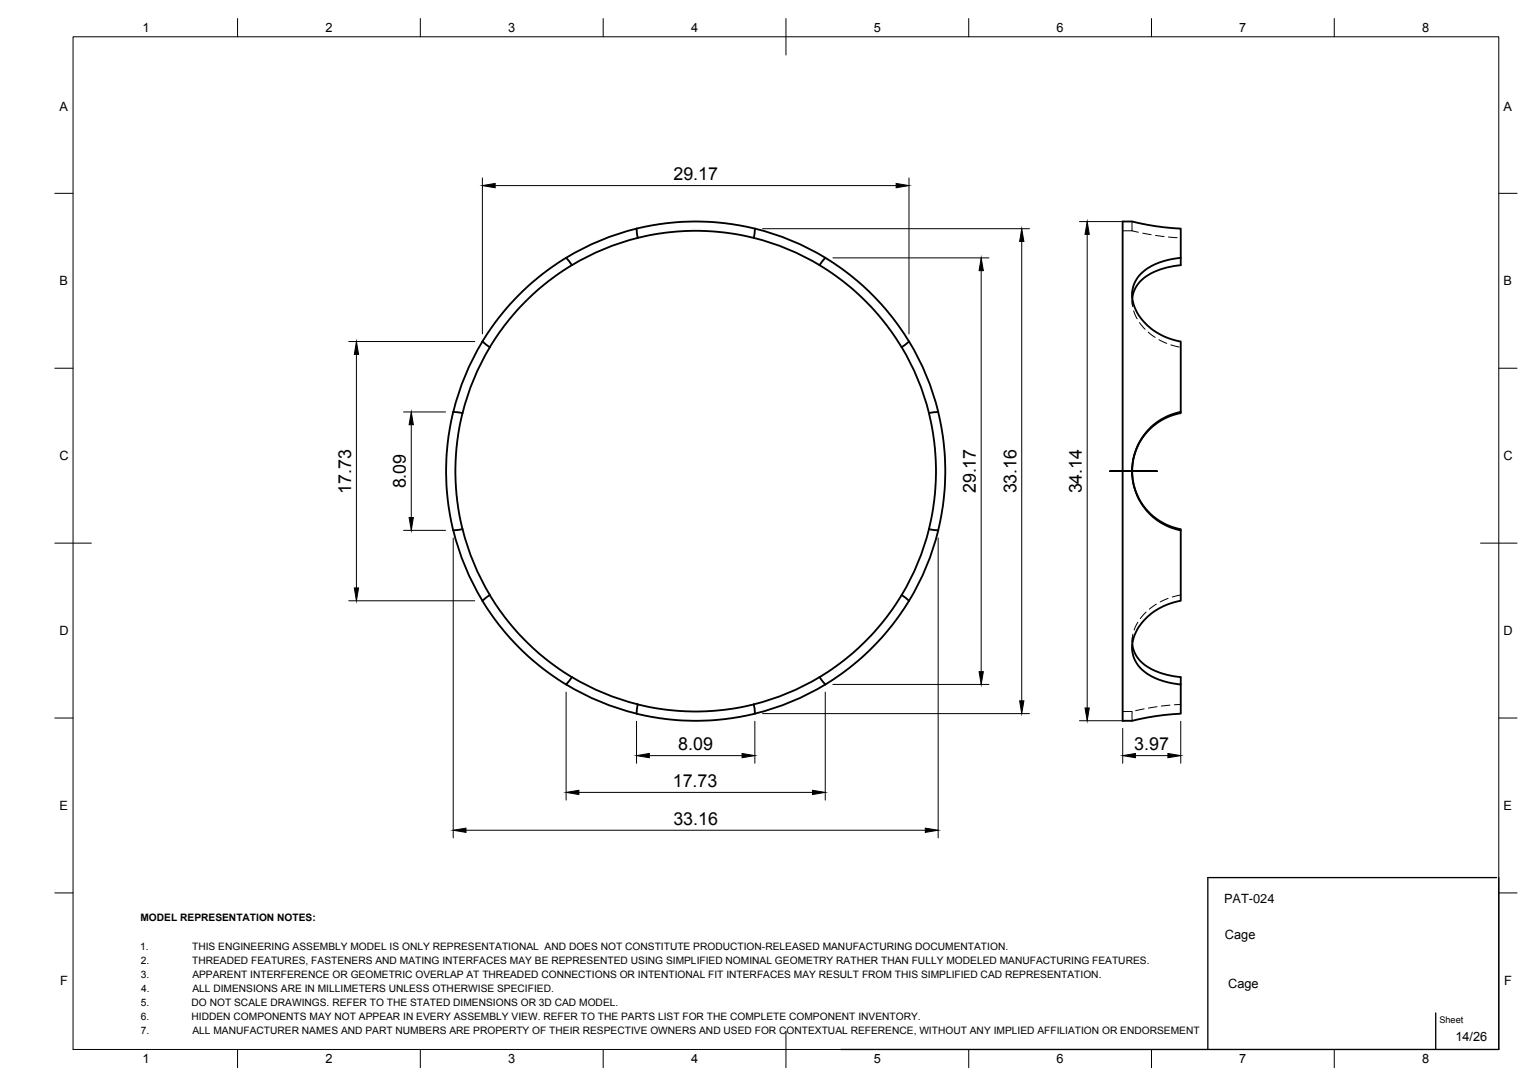
ISO-10303-21;
HEADER;
/* Generated by software containing ST-Developer
 * from STEP Tools, Inc. (www.steptools.com) 
 */

FILE_DESCRIPTION(
/* description */ ('Compact handwheel screw vise'),
/* implementation_level */ '2;1');

FILE_NAME(
/* name */ 'Cage.step',
/* time_stamp */ '2026-10-29T16:08:22-07:00',
/* author */ (''),
/* organization */ (''),
/* preprocessor_version */ 'ST-DEVELOPER v20.2',
/* originating_system */ 'Autodesk Translation Framework v15.17.0.0',
/* authorisation */ '');

FILE_SCHEMA (('AUTOMOTIVE_DESIGN { 1 0 10303 214 3 1 1 }'));
ENDSEC;

DATA;
#10=MECHANICAL_DESIGN_GEOMETRIC_PRESENTATION_REPRESENTATION('',(#661),#25074);
#211=B_SPLINE_CURVE_WITH_KNOTS('',3,(#11837,#11838,#11839,#11840,#11841,
#11842,#11843,#11844,#11845,#11846,#11847,#11848,#11849,#11850,#11851,#11852,
#11853,#11854,#11855,#11856,#11857,#11858),.UNSPECIFIED.,.F.,.F.,(4,2,2,
2,2,2,2,2,2,2,4),(0.0789094028588958,0.210573405340968,0.315860108011452,
0.421146810681936,0.522142632548711,0.623138454415485,0.72413427628226,
0.825130098149035,0.930416800819519,1.03570350349,1.16736750597208),
 .UNSPECIFIED.);
#212=B_SPLINE_CURVE_WITH_KNOTS('',3,(#11862,#11863,#11864,#11865,#11866,
#11867,#11868,#11869,#11870,#11871,#11872,#11873,#11874,#11875,#11876,#11877,
#11878,#11879,#11880,#11881,#11882,#11883),.UNSPECIFIED.,.F.,.F.,(4,2,2,
2,2,2,2,2,2,2,4),(0.0774793363974613,0.142088896491891,0.284177792983782,
0.411119756996526,0.514392970548519,0.617666184100513,0.720939397652506,
0.8242126112045,0.951154575217244,1.09324347170913,1.15785303180356),
 .UNSPECIFIED.);
#213=B_SPLINE_CURVE_WITH_KNOTS('',3,(#11889,#11890,#11891,#11892,#11893,
#11894,#11895,#11896,#11897,#11898,#11899,#11900,#11901,#11902,#11903,#11904,
#11905,#11906,#11907,#11908,#11909,#11910),.UNSPECIFIED.,.F.,.F.,(4,2,2,
2,2,2,2,2,2,2,4),(0.0774793363974613,0.142088896491891,0.284177792983782,
0.411119756996525,0.514392970548519,0.617666184100513,0.720939397652506,
0.8242126112045,0.951154575217243,1.09324347170913,1.15785303180356),
 .UNSPECIFIED.);
#214=B_SPLINE_CURVE_WITH_KNOTS('',3,(#11914,#11915,#11916,#11917,#11918,
#11919,#11920,#11921,#11922,#11923,#11924,#11925,#11926,#11927,#11928,#11929,
#11930,#11931,#11932,#11933,#11934,#11935),.UNSPECIFIED.,.F.,.F.,(4,2,2,
2,2,2,2,2,2,2,4),(0.0774793363974614,0.142088896491891,0.284177792983781,
0.411119756996525,0.514392970548519,0.617666184100512,0.720939397652506,
0.824212611204499,0.951154575217243,1.09324347170913,1.15785303180356),
 .UNSPECIFIED.);
#215=B_SPLINE_CURVE_WITH_KNOTS('',3,(#11939,#11940,#11941,#11942,#11943,
#11944,#11945,#11946,#11947,#11948,#11949,#11950),.UNSPECIFIED.,.F.,.F.,
(4,2,2,2,2,4),(0.0774793363974613,0.142088896491891,0.284177792983781,0.411119756996525,
0.514392970548519,0.617666184100512),.UNSPECIFIED.);
#216=B_SPLINE_CURVE_WITH_KNOTS('',3,(#11955,#11956,#11957,#11958,#11959,
#11960,#11961,#11962,#11963,#11964,#11965,#11966),.UNSPECIFIED.,.F.,.F.,
(4,2,2,2,2,4),(0.617666184100512,0.720939397652506,0.824212611204499,0.951154575217243,
1.09324347170913,1.15785303180356),.UNSPECIFIED.);
#217=B_SPLINE_CURVE_WITH_KNOTS('',3,(#11970,#11971,#11972,#11973,#11974,
#11975,#11976,#11977,#11978,#11979,#11980,#11981,#11982,#11983,#11984,#11985,
#11986,#11987,#11988,#11989,#11990,#11991),.UNSPECIFIED.,.F.,.F.,(4,2,2,
2,2,2,2,2,2,2,4),(0.0774793363974613,0.142088896491891,0.284177792983782,
0.411119756996526,0.514392970548519,0.617666184100513,0.720939397652507,
0.8242126112045,0.951154575217245,1.09324347170914,1.15785303180356),
 .UNSPECIFIED.);
#218=B_SPLINE_CURVE_WITH_KNOTS('',3,(#11995,#11996,#11997,#11998,#11999,
#12000,#12001,#12002,#12003,#12004,#12005,#12006,#12007,#12008,#12009,#12010,
#12011,#12012,#12013,#12014,#12015,#12016),.UNSPECIFIED.,.F.,.F.,(4,2,2,
2,2,2,2,2,2,2,4),(0.0774793363974613,0.142088896491891,0.284177792983782,
0.411119756996526,0.514392970548519,0.617666184100513,0.720939397652506,
0.824212611204499,0.951154575217243,1.09324347170913,1.15785303180356),
 .UNSPECIFIED.);
#219=B_SPLINE_CURVE_WITH_KNOTS('',3,(#12020,#12021,#12022,#12023,#12024,
#12025,#12026,#12027,#12028,#12029,#12030,#12031,#12032,#12033,#12034,#12035,
#12036,#12037,#12038,#12039,#12040,#12041),.UNSPECIFIED.,.F.,.F.,(4,2,2,
2,2,2,2,2,2,2,4),(0.0774793363974613,0.142088896491891,0.284177792983782,
0.411119756996526,0.514392970548519,0.617666184100513,0.720939397652506,
0.8242126112045,0.951154575217244,1.09324347170913,1.15785303180356),
 .UNSPECIFIED.);
#220=B_SPLINE_CURVE_WITH_KNOTS('',3,(#12045,#12046,#12047,#12048,#12049,
#12050,#12051,#12052,#12053,#12054,#12055,#12056,#12057,#12058,#12059,#12060,
#12061,#12062,#12063,#12064,#12065,#12066),.UNSPECIFIED.,.F.,.F.,(4,2,2,
2,2,2,2,2,2,2,4),(0.0774793363974613,0.142088896491891,0.284177792983782,
0.411119756996526,0.514392970548519,0.617666184100513,0.720939397652506,
0.8242126112045,0.951154575217243,1.09324347170913,1.15785303180356),
 .UNSPECIFIED.);
#221=B_SPLINE_CURVE_WITH_KNOTS('',3,(#12074,#12075,#12076,#12077,#12078,
#12079,#12080,#12081,#12082,#12083,#12084,#12085,#12086,#12087,#12088,#12089,
#12090,#12091,#12092,#12093,#12094,#12095),.UNSPECIFIED.,.F.,.F.,(4,2,2,
2,2,2,2,2,2,2,4),(0.0789094028588958,0.210573405340968,0.315860108011452,
0.421146810681936,0.522142632548711,0.623138454415485,0.72413427628226,
0.825130098149035,0.930416800819519,1.03570350349,1.16736750597208),
 .UNSPECIFIED.);
#222=B_SPLINE_CURVE_WITH_KNOTS('',3,(#12103,#12104,#12105,#12106,#12107,
#12108,#12109,#12110,#12111,#12112,#12113,#12114,#12115,#12116,#12117,#12118,
#12119,#12120,#12121,#12122,#12123,#12124),.UNSPECIFIED.,.F.,.F.,(4,2,2,
2,2,2,2,2,2,2,4),(0.0789094028588958,0.210573405340969,0.315860108011453,
0.421146810681937,0.522142632548712,0.623138454415486,0.724134276282261,
0.825130098149035,0.930416800819519,1.03570350349,1.16736750597208),
 .UNSPECIFIED.);
#223=B_SPLINE_CURVE_WITH_KNOTS('',3,(#12133,#12134,#12135,#12136,#12137,
#12138,#12139,#12140,#12141,#12142,#12143,#12144),.UNSPECIFIED.,.F.,.F.,
(4,2,2,2,2,4),(0.0789094028588958,0.210573405340968,0.315860108011452,0.421146810681937,
0.522142632548711,0.623138454415486),.UNSPECIFIED.);
#224=B_SPLINE_CURVE_WITH_KNOTS('',3,(#12146,#12147,#12148,#12149,#12150,
#12151,#12152,#12153,#12154,#12155,#12156,#12157),.UNSPECIFIED.,.F.,.F.,
(4,2,2,2,2,4),(0.623138454415486,0.72413427628226,0.825130098149035,0.930416800819519,
1.03570350349,1.16736750597208),.UNSPECIFIED.);
#225=B_SPLINE_CURVE_WITH_KNOTS('',3,(#12164,#12165,#12166,#12167,#12168,
#12169,#12170,#12171,#12172,#12173,#12174,#12175,#12176,#12177,#12178,#12179,
#12180,#12181,#12182,#12183,#12184,#12185),.UNSPECIFIED.,.F.,.F.,(4,2,2,
2,2,2,2,2,2,2,4),(0.0789094028588958,0.210573405340968,0.315860108011452,
0.421146810681936,0.522142632548711,0.623138454415486,0.72413427628226,
0.825130098149035,0.930416800819519,1.03570350349,1.16736750597208),
 .UNSPECIFIED.);
#226=B_SPLINE_CURVE_WITH_KNOTS('',3,(#12193,#12194,#12195,#12196,#12197,
#12198,#12199,#12200,#12201,#12202,#12203,#12204,#12205,#12206,#12207,#12208,
#12209,#12210,#12211,#12212,#12213,#12214),.UNSPECIFIED.,.F.,.F.,(4,2,2,
2,2,2,2,2,2,2,4),(0.0789094028588957,0.210573405340968,0.315860108011452,
0.421146810681936,0.522142632548711,0.623138454415485,0.72413427628226,
0.825130098149035,0.930416800819519,1.03570350349,1.16736750597207),
 .UNSPECIFIED.);
#227=B_SPLINE_CURVE_WITH_KNOTS('',3,(#12222,#12223,#12224,#12225,#12226,
#12227,#12228,#12229,#12230,#12231,#12232,#12233,#12234,#12235,#12236,#12237,
#12238,#12239,#12240,#12241,#12242,#12243),.UNSPECIFIED.,.F.,.F.,(4,2,2,
2,2,2,2,2,2,2,4),(0.0789094028588958,0.210573405340968,0.315860108011452,
0.421146810681936,0.522142632548711,0.623138454415486,0.72413427628226,
0.825130098149035,0.930416800819519,1.03570350349,1.16736750597208),
 .UNSPECIFIED.);
#228=B_SPLINE_CURVE_WITH_KNOTS('',3,(#12252,#12253,#12254,#12255,#12256,
#12257,#12258,#12259,#12260,#12261,#12262,#12263,#12264,#12265,#12266,#12267,
#12268,#12269,#12270,#12271,#12272,#12273),.UNSPECIFIED.,.F.,.F.,(4,2,2,
2,2,2,2,2,2,2,4),(0.0789094028588958,0.210573405340968,0.315860108011452,
0.421146810681936,0.522142632548711,0.623138454415485,0.72413427628226,
0.825130098149035,0.930416800819519,1.03570350349,1.16736750597208),
 .UNSPECIFIED.);
#549=SPHERICAL_SURFACE('',#8631,0.412776);
#550=SPHERICAL_SURFACE('',#8647,0.412776);
#551=SPHERICAL_SURFACE('',#8652,0.412776);
#552=SPHERICAL_SURFACE('',#8657,0.412776);
#553=SPHERICAL_SURFACE('',#8662,0.412776);
#554=SPHERICAL_SURFACE('',#8667,0.412776);
#555=SPHERICAL_SURFACE('',#8672,0.412776);
#556=SPHERICAL_SURFACE('',#8680,0.412776);
#598=SHAPE_REPRESENTATION_RELATIONSHIP('SRR','None',#25207,#626);
#626=ADVANCED_BREP_SHAPE_REPRESENTATION('',(#696),#25054);
#661=STYLED_ITEM('',(#25439),#696);
#696=MANIFOLD_SOLID_BREP('Continuous crown cage',#8070);
#764=FACE_BOUND('',#1669,.T.);
#883=PLANE('',#8644);
#884=PLANE('',#8649);
#885=PLANE('',#8654);
#886=PLANE('',#8659);
#887=PLANE('',#8664);
#888=PLANE('',#8669);
#889=PLANE('',#8678);
#890=PLANE('',#8682);
#891=PLANE('',#8683);
#1129=FACE_OUTER_BOUND('',#1651,.T.);
#1130=FACE_OUTER_BOUND('',#1652,.T.);
#1131=FACE_OUTER_BOUND('',#1653,.T.);
#1132=FACE_OUTER_BOUND('',#1654,.T.);
#1133=FACE_OUTER_BOUND('',#1655,.T.);
#1134=FACE_OUTER_BOUND('',#1656,.T.);
#1135=FACE_OUTER_BOUND('',#1657,.T.);
#1136=FACE_OUTER_BOUND('',#1658,.T.);
#1137=FACE_OUTER_BOUND('',#1659,.T.);
#1138=FACE_OUTER_BOUND('',#1660,.T.);
#1139=FACE_OUTER_BOUND('',#1661,.T.);
#1140=FACE_OUTER_BOUND('',#1662,.T.);
#1141=FACE_OUTER_BOUND('',#1663,.T.);
#1142=FACE_OUTER_BOUND('',#1664,.T.);
#1143=FACE_OUTER_BOUND('',#1665,.T.);
#1144=FACE_OUTER_BOUND('',#1666,.T.);
#1145=FACE_OUTER_BOUND('',#1667,.T.);
#1146=FACE_OUTER_BOUND('',#1668,.T.);
#1147=FACE_OUTER_BOUND('',#1670,.T.);
#1651=EDGE_LOOP('',(#5611,#5612,#5613,#5614));
#1652=EDGE_LOOP('',(#5615,#5616,#5617,#5618,#5619,#5620,#5621,#5622,#5623,
#5624,#5625,#5626,#5627,#5628,#5629,#5630,#5631,#5632,#5633,#5634));
#1653=EDGE_LOOP('',(#5635,#5636,#5637,#5638));
#1654=EDGE_LOOP('',(#5639,#5640,#5641,#5642));
#1655=EDGE_LOOP('',(#5643,#5644,#5645,#5646));
#1656=EDGE_LOOP('',(#5647,#5648,#5649,#5650));
#1657=EDGE_LOOP('',(#5651,#5652,#5653,#5654));
#1658=EDGE_LOOP('',(#5655,#5656,#5657,#5658,#5659,#5660));
#1659=EDGE_LOOP('',(#5661,#5662,#5663,#5664));
#1660=EDGE_LOOP('',(#5665,#5666,#5667,#5668));
#1661=EDGE_LOOP('',(#5669,#5670,#5671,#5672));
#1662=EDGE_LOOP('',(#5673,#5674,#5675,#5676));
#1663=EDGE_LOOP('',(#5677,#5678,#5679,#5680));
#1664=EDGE_LOOP('',(#5681,#5682,#5683,#5684));
#1665=EDGE_LOOP('',(#5685,#5686,#5687,#5688,#5689,#5690,#5691,#5692,#5693,
#5694,#5695,#5696,#5697,#5698,#5699,#5700,#5701,#5702,#5703,#5704));
#1666=EDGE_LOOP('',(#5705,#5706,#5707,#5708));
#1667=EDGE_LOOP('',(#5709,#5710,#5711,#5712));
#1668=EDGE_LOOP('',(#5713));
#1669=EDGE_LOOP('',(#5714));
#1670=EDGE_LOOP('',(#5715,#5716,#5717,#5718));
#2189=LINE('',#11952,#2697);
#2190=LINE('',#12248,#2698);
#2697=VECTOR('',#9805,1.706752);
#2698=VECTOR('',#9882,1.643248);
#3177=CIRCLE('',#8632,0.405071403305639);
#3178=CIRCLE('',#8633,0.405071403305639);
#3179=CIRCLE('',#8635,1.706752);
#3180=CIRCLE('',#8636,1.706752);
#3181=CIRCLE('',#8637,1.706752);
#3182=CIRCLE('',#8638,1.706752);
#3183=CIRCLE('',#8639,1.706752);
#3184=CIRCLE('',#8640,1.706752);
#3185=CIRCLE('',#8641,1.706752);
#3186=CIRCLE('',#8642,1.706752);
#3187=CIRCLE('',#8643,1.706752);
#3188=CIRCLE('',#8645,1.643248);
#3189=CIRCLE('',#8646,0.405071403305639);
#3190=CIRCLE('',#8648,0.405071403305639);
#3191=CIRCLE('',#8650,1.643248);
#3192=CIRCLE('',#8651,0.405071403305639);
#3193=CIRCLE('',#8653,0.405071403305639);
#3194=CIRCLE('',#8655,1.643248);
#3195=CIRCLE('',#8656,0.405071403305639);
#3196=CIRCLE('',#8658,0.405071403305639);
#3197=CIRCLE('',#8660,1.643248);
#3198=CIRCLE('',#8661,0.405071403305639);
#3199=CIRCLE('',#8663,0.405071403305639);
#3200=CIRCLE('',#8665,1.643248);
#3201=CIRCLE('',#8666,0.405071403305639);
#3202=CIRCLE('',#8668,0.405071403305639);
#3203=CIRCLE('',#8670,1.643248);
#3204=CIRCLE('',#8671,0.405071403305639);
#3205=CIRCLE('',#8673,0.405071403305639);
#3206=CIRCLE('',#8675,1.643248);
#3207=CIRCLE('',#8676,1.643248);
#3208=CIRCLE('',#8677,1.643248);
#3209=CIRCLE('',#8679,0.405071403305639);
#3210=CIRCLE('',#8681,0.405071403305639);
#3492=VERTEX_POINT('',#11835);
#3493=VERTEX_POINT('',#11836);
#3494=VERTEX_POINT('',#11859);
#3495=VERTEX_POINT('',#11861);
#3496=VERTEX_POINT('',#11886);
#3497=VERTEX_POINT('',#11888);
#3498=VERTEX_POINT('',#11911);
#3499=VERTEX_POINT('',#11913);
#3500=VERTEX_POINT('',#11936);
#3501=VERTEX_POINT('',#11938);
#3502=VERTEX_POINT('',#11951);
#3503=VERTEX_POINT('',#11954);
#3504=VERTEX_POINT('',#11967);
#3505=VERTEX_POINT('',#11969);
#3506=VERTEX_POINT('',#11992);
#3507=VERTEX_POINT('',#11994);
#3508=VERTEX_POINT('',#12017);
#3509=VERTEX_POINT('',#12019);
#3510=VERTEX_POINT('',#12042);
#3511=VERTEX_POINT('',#12044);
#3512=VERTEX_POINT('',#12069);
#3513=VERTEX_POINT('',#12073);
#3514=VERTEX_POINT('',#12098);
#3515=VERTEX_POINT('',#12102);
#3516=VERTEX_POINT('',#12127);
#3517=VERTEX_POINT('',#12131);
#3518=VERTEX_POINT('',#12132);
#3519=VERTEX_POINT('',#12159);
#3520=VERTEX_POINT('',#12163);
#3521=VERTEX_POINT('',#12188);
#3522=VERTEX_POINT('',#12192);
#3523=VERTEX_POINT('',#12217);
#3524=VERTEX_POINT('',#12221);
#3525=VERTEX_POINT('',#12246);
#3526=VERTEX_POINT('',#12249);
#3527=VERTEX_POINT('',#12251);
#4292=EDGE_CURVE('',#3492,#3493,#211,.T.);
#4293=EDGE_CURVE('',#3494,#3492,#3177,.T.);
#4294=EDGE_CURVE('',#3495,#3494,#212,.T.);
#4295=EDGE_CURVE('',#3493,#3495,#3178,.T.);
#4296=EDGE_CURVE('',#3496,#3494,#3179,.T.);
#4297=EDGE_CURVE('',#3496,#3497,#213,.T.);
#4298=EDGE_CURVE('',#3498,#3497,#3180,.T.);
#4299=EDGE_CURVE('',#3498,#3499,#214,.T.);
#4300=EDGE_CURVE('',#3500,#3499,#3181,.T.);
#4301=EDGE_CURVE('',#3500,#3501,#215,.T.);
#4302=EDGE_CURVE('',#3501,#3502,#2189,.T.);
#4303=EDGE_CURVE('',#3502,#3502,#3182,.T.);
#4304=EDGE_CURVE('',#3501,#3503,#216,.T.);
#4305=EDGE_CURVE('',#3504,#3503,#3183,.T.);
#4306=EDGE_CURVE('',#3504,#3505,#217,.T.);
#4307=EDGE_CURVE('',#3506,#3505,#3184,.T.);
#4308=EDGE_CURVE('',#3506,#3507,#218,.T.);
#4309=EDGE_CURVE('',#3508,#3507,#3185,.T.);
#4310=EDGE_CURVE('',#3508,#3509,#219,.T.);
#4311=EDGE_CURVE('',#3510,#3509,#3186,.T.);
#4312=EDGE_CURVE('',#3510,#3511,#220,.T.);
#4313=EDGE_CURVE('',#3495,#3511,#3187,.T.);
#4314=EDGE_CURVE('',#3492,#3512,#3188,.T.);
#4315=EDGE_CURVE('',#3512,#3496,#3189,.T.);
#4316=EDGE_CURVE('',#3513,#3512,#221,.T.);
#4317=EDGE_CURVE('',#3497,#3513,#3190,.T.);
#4318=EDGE_CURVE('',#3513,#3514,#3191,.T.);
#4319=EDGE_CURVE('',#3514,#3498,#3192,.T.);
#4320=EDGE_CURVE('',#3515,#3514,#222,.T.);
#4321=EDGE_CURVE('',#3499,#3515,#3193,.T.);
#4322=EDGE_CURVE('',#3515,#3516,#3194,.T.);
#4323=EDGE_CURVE('',#3516,#3500,#3195,.T.);
#4324=EDGE_CURVE('',#3517,#3518,#223,.T.);
#4325=EDGE_CURVE('',#3503,#3517,#3196,.T.);
#4326=EDGE_CURVE('',#3518,#3516,#224,.T.);
#4327=EDGE_CURVE('',#3517,#3519,#3197,.T.);
#4328=EDGE_CURVE('',#3519,#3504,#3198,.T.);
#4329=EDGE_CURVE('',#3520,#3519,#225,.T.);
#4330=EDGE_CURVE('',#3505,#3520,#3199,.T.);
#4331=EDGE_CURVE('',#3520,#3521,#3200,.T.);
#4332=EDGE_CURVE('',#3521,#3506,#3201,.T.);
#4333=EDGE_CURVE('',#3522,#3521,#226,.T.);
#4334=EDGE_CURVE('',#3507,#3522,#3202,.T.);
#4335=EDGE_CURVE('',#3522,#3523,#3203,.T.);
#4336=EDGE_CURVE('',#3523,#3508,#3204,.T.);
#4337=EDGE_CURVE('',#3524,#3523,#227,.T.);
#4338=EDGE_CURVE('',#3509,#3524,#3205,.T.);
#4339=EDGE_CURVE('',#3525,#3525,#3206,.T.);
#4340=EDGE_CURVE('',#3525,#3518,#2190,.T.);
#4341=EDGE_CURVE('',#3526,#3493,#3207,.T.);
#4342=EDGE_CURVE('',#3526,#3527,#228,.T.);
#4343=EDGE_CURVE('',#3524,#3527,#3208,.T.);
#4344=EDGE_CURVE('',#3511,#3526,#3209,.T.);
#4345=EDGE_CURVE('',#3527,#3510,#3210,.T.);
#5611=ORIENTED_EDGE('',*,*,#4292,.F.);
#5612=ORIENTED_EDGE('',*,*,#4293,.F.);
#5613=ORIENTED_EDGE('',*,*,#4294,.F.);
#5614=ORIENTED_EDGE('',*,*,#4295,.F.);
#5615=ORIENTED_EDGE('',*,*,#4294,.T.);
#5616=ORIENTED_EDGE('',*,*,#4296,.F.);
#5617=ORIENTED_EDGE('',*,*,#4297,.T.);
#5618=ORIENTED_EDGE('',*,*,#4298,.F.);
#5619=ORIENTED_EDGE('',*,*,#4299,.T.);
#5620=ORIENTED_EDGE('',*,*,#4300,.F.);
#5621=ORIENTED_EDGE('',*,*,#4301,.T.);
#5622=ORIENTED_EDGE('',*,*,#4302,.T.);
#5623=ORIENTED_EDGE('',*,*,#4303,.F.);
#5624=ORIENTED_EDGE('',*,*,#4302,.F.);
#5625=ORIENTED_EDGE('',*,*,#4304,.T.);
#5626=ORIENTED_EDGE('',*,*,#4305,.F.);
#5627=ORIENTED_EDGE('',*,*,#4306,.T.);
#5628=ORIENTED_EDGE('',*,*,#4307,.F.);
#5629=ORIENTED_EDGE('',*,*,#4308,.T.);
#5630=ORIENTED_EDGE('',*,*,#4309,.F.);
#5631=ORIENTED_EDGE('',*,*,#4310,.T.);
#5632=ORIENTED_EDGE('',*,*,#4311,.F.);
#5633=ORIENTED_EDGE('',*,*,#4312,.T.);
#5634=ORIENTED_EDGE('',*,*,#4313,.F.);
#5635=ORIENTED_EDGE('',*,*,#4293,.T.);
#5636=ORIENTED_EDGE('',*,*,#4314,.T.);
#5637=ORIENTED_EDGE('',*,*,#4315,.T.);
#5638=ORIENTED_EDGE('',*,*,#4296,.T.);
#5639=ORIENTED_EDGE('',*,*,#4316,.F.);
#5640=ORIENTED_EDGE('',*,*,#4317,.F.);
#5641=ORIENTED_EDGE('',*,*,#4297,.F.);
#5642=ORIENTED_EDGE('',*,*,#4315,.F.);
#5643=ORIENTED_EDGE('',*,*,#4317,.T.);
#5644=ORIENTED_EDGE('',*,*,#4318,.T.);
#5645=ORIENTED_EDGE('',*,*,#4319,.T.);
#5646=ORIENTED_EDGE('',*,*,#4298,.T.);
#5647=ORIENTED_EDGE('',*,*,#4320,.F.);
#5648=ORIENTED_EDGE('',*,*,#4321,.F.);
#5649=ORIENTED_EDGE('',*,*,#4299,.F.);
#5650=ORIENTED_EDGE('',*,*,#4319,.F.);
#5651=ORIENTED_EDGE('',*,*,#4321,.T.);
#5652=ORIENTED_EDGE('',*,*,#4322,.T.);
#5653=ORIENTED_EDGE('',*,*,#4323,.T.);
#5654=ORIENTED_EDGE('',*,*,#4300,.T.);
#5655=ORIENTED_EDGE('',*,*,#4324,.F.);
#5656=ORIENTED_EDGE('',*,*,#4325,.F.);
#5657=ORIENTED_EDGE('',*,*,#4304,.F.);
#5658=ORIENTED_EDGE('',*,*,#4301,.F.);
#5659=ORIENTED_EDGE('',*,*,#4323,.F.);
#5660=ORIENTED_EDGE('',*,*,#4326,.F.);
#5661=ORIENTED_EDGE('',*,*,#4325,.T.);
#5662=ORIENTED_EDGE('',*,*,#4327,.T.);
#5663=ORIENTED_EDGE('',*,*,#4328,.T.);
#5664=ORIENTED_EDGE('',*,*,#4305,.T.);
#5665=ORIENTED_EDGE('',*,*,#4329,.F.);
#5666=ORIENTED_EDGE('',*,*,#4330,.F.);
#5667=ORIENTED_EDGE('',*,*,#4306,.F.);
#5668=ORIENTED_EDGE('',*,*,#4328,.F.);
#5669=ORIENTED_EDGE('',*,*,#4330,.T.);
#5670=ORIENTED_EDGE('',*,*,#4331,.T.);
#5671=ORIENTED_EDGE('',*,*,#4332,.T.);
#5672=ORIENTED_EDGE('',*,*,#4307,.T.);
#5673=ORIENTED_EDGE('',*,*,#4333,.F.);
#5674=ORIENTED_EDGE('',*,*,#4334,.F.);
#5675=ORIENTED_EDGE('',*,*,#4308,.F.);
#5676=ORIENTED_EDGE('',*,*,#4332,.F.);
#5677=ORIENTED_EDGE('',*,*,#4334,.T.);
#5678=ORIENTED_EDGE('',*,*,#4335,.T.);
#5679=ORIENTED_EDGE('',*,*,#4336,.T.);
#5680=ORIENTED_EDGE('',*,*,#4309,.T.);
#5681=ORIENTED_EDGE('',*,*,#4310,.F.);
#5682=ORIENTED_EDGE('',*,*,#4336,.F.);
#5683=ORIENTED_EDGE('',*,*,#4337,.F.);
#5684=ORIENTED_EDGE('',*,*,#4338,.F.);
#5685=ORIENTED_EDGE('',*,*,#4339,.F.);
#5686=ORIENTED_EDGE('',*,*,#4340,.T.);
#5687=ORIENTED_EDGE('',*,*,#4326,.T.);
#5688=ORIENTED_EDGE('',*,*,#4322,.F.);
#5689=ORIENTED_EDGE('',*,*,#4320,.T.);
#5690=ORIENTED_EDGE('',*,*,#4318,.F.);
#5691=ORIENTED_EDGE('',*,*,#4316,.T.);
#5692=ORIENTED_EDGE('',*,*,#4314,.F.);
#5693=ORIENTED_EDGE('',*,*,#4292,.T.);
#5694=ORIENTED_EDGE('',*,*,#4341,.F.);
#5695=ORIENTED_EDGE('',*,*,#4342,.T.);
#5696=ORIENTED_EDGE('',*,*,#4343,.F.);
#5697=ORIENTED_EDGE('',*,*,#4337,.T.);
#5698=ORIENTED_EDGE('',*,*,#4335,.F.);
#5699=ORIENTED_EDGE('',*,*,#4333,.T.);
#5700=ORIENTED_EDGE('',*,*,#4331,.F.);
#5701=ORIENTED_EDGE('',*,*,#4329,.T.);
#5702=ORIENTED_EDGE('',*,*,#4327,.F.);
#5703=ORIENTED_EDGE('',*,*,#4324,.T.);
#5704=ORIENTED_EDGE('',*,*,#4340,.F.);
#5705=ORIENTED_EDGE('',*,*,#4295,.T.);
#5706=ORIENTED_EDGE('',*,*,#4313,.T.);
#5707=ORIENTED_EDGE('',*,*,#4344,.T.);
#5708=ORIENTED_EDGE('',*,*,#4341,.T.);
#5709=ORIENTED_EDGE('',*,*,#4312,.F.);
#5710=ORIENTED_EDGE('',*,*,#4345,.F.);
#5711=ORIENTED_EDGE('',*,*,#4342,.F.);
#5712=ORIENTED_EDGE('',*,*,#4344,.F.);
#5713=ORIENTED_EDGE('',*,*,#4303,.T.);
#5714=ORIENTED_EDGE('',*,*,#4339,.T.);
#5715=ORIENTED_EDGE('',*,*,#4338,.T.);
#5716=ORIENTED_EDGE('',*,*,#4343,.T.);
#5717=ORIENTED_EDGE('',*,*,#4345,.T.);
#5718=ORIENTED_EDGE('',*,*,#4311,.T.);
#7384=CYLINDRICAL_SURFACE('',#8634,1.706752);
#7385=CYLINDRICAL_SURFACE('',#8674,1.643248);
#7699=ADVANCED_FACE('',(#1129),#549,.F.);
#7700=ADVANCED_FACE('',(#1130),#7384,.T.);
#7701=ADVANCED_FACE('',(#1131),#883,.T.);
#7702=ADVANCED_FACE('',(#1132),#550,.F.);
#7703=ADVANCED_FACE('',(#1133),#884,.T.);
#7704=ADVANCED_FACE('',(#1134),#551,.F.);
#7705=ADVANCED_FACE('',(#1135),#885,.T.);
#7706=ADVANCED_FACE('',(#1136),#552,.F.);
#7707=ADVANCED_FACE('',(#1137),#886,.T.);
#7708=ADVANCED_FACE('',(#1138),#553,.F.);
#7709=ADVANCED_FACE('',(#1139),#887,.T.);
#7710=ADVANCED_FACE('',(#1140),#554,.F.);
#7711=ADVANCED_FACE('',(#1141),#888,.T.);
#7712=ADVANCED_FACE('',(#1142),#555,.F.);
#7713=ADVANCED_FACE('',(#1143),#7385,.F.);
#7714=ADVANCED_FACE('',(#1144),#889,.T.);
#7715=ADVANCED_FACE('',(#1145),#556,.F.);
#7716=ADVANCED_FACE('',(#1146,#764),#890,.T.);
#7717=ADVANCED_FACE('',(#1147),#891,.T.);
#8070=CLOSED_SHELL('',(#7699,#7700,#7701,#7702,#7703,#7704,#7705,#7706,
#7707,#7708,#7709,#7710,#7711,#7712,#7713,#7714,#7715,#7716,#7717));
#8630=AXIS2_PLACEMENT_3D('',#11833,#9789,#9790);
#8631=AXIS2_PLACEMENT_3D('',#11834,#9791,#9792);
#8632=AXIS2_PLACEMENT_3D('',#11860,#9793,#9794);
#8633=AXIS2_PLACEMENT_3D('',#11884,#9795,#9796);
#8634=AXIS2_PLACEMENT_3D('',#11885,#9797,#9798);
#8635=AXIS2_PLACEMENT_3D('',#11887,#9799,#9800);
#8636=AXIS2_PLACEMENT_3D('',#11912,#9801,#9802);
#8637=AXIS2_PLACEMENT_3D('',#11937,#9803,#9804);
#8638=AXIS2_PLACEMENT_3D('',#11953,#9806,#9807);
#8639=AXIS2_PLACEMENT_3D('',#11968,#9808,#9809);
#8640=AXIS2_PLACEMENT_3D('',#11993,#9810,#9811);
#8641=AXIS2_PLACEMENT_3D('',#12018,#9812,#9813);
#8642=AXIS2_PLACEMENT_3D('',#12043,#9814,#9815);
#8643=AXIS2_PLACEMENT_3D('',#12067,#9816,#9817);
#8644=AXIS2_PLACEMENT_3D('',#12068,#9818,#9819);
#8645=AXIS2_PLACEMENT_3D('',#12070,#9820,#9821);
#8646=AXIS2_PLACEMENT_3D('',#12071,#9822,#9823);
#8647=AXIS2_PLACEMENT_3D('',#12072,#9824,#9825);
#8648=AXIS2_PLACEMENT_3D('',#12096,#9826,#9827);
#8649=AXIS2_PLACEMENT_3D('',#12097,#9828,#9829);
#8650=AXIS2_PLACEMENT_3D('',#12099,#9830,#9831);
#8651=AXIS2_PLACEMENT_3D('',#12100,#9832,#9833);
#8652=AXIS2_PLACEMENT_3D('',#12101,#9834,#9835);
#8653=AXIS2_PLACEMENT_3D('',#12125,#9836,#9837);
#8654=AXIS2_PLACEMENT_3D('',#12126,#9838,#9839);
#8655=AXIS2_PLACEMENT_3D('',#12128,#9840,#9841);
#8656=AXIS2_PLACEMENT_3D('',#12129,#9842,#9843);
#8657=AXIS2_PLACEMENT_3D('',#12130,#9844,#9845);
#8658=AXIS2_PLACEMENT_3D('',#12145,#9846,#9847);
#8659=AXIS2_PLACEMENT_3D('',#12158,#9848,#9849);
#8660=AXIS2_PLACEMENT_3D('',#12160,#9850,#9851);
#8661=AXIS2_PLACEMENT_3D('',#12161,#9852,#9853);
#8662=AXIS2_PLACEMENT_3D('',#12162,#9854,#9855);
#8663=AXIS2_PLACEMENT_3D('',#12186,#9856,#9857);
#8664=AXIS2_PLACEMENT_3D('',#12187,#9858,#9859);
#8665=AXIS2_PLACEMENT_3D('',#12189,#9860,#9861);
#8666=AXIS2_PLACEMENT_3D('',#12190,#9862,#9863);
#8667=AXIS2_PLACEMENT_3D('',#12191,#9864,#9865);
#8668=AXIS2_PLACEMENT_3D('',#12215,#9866,#9867);
#8669=AXIS2_PLACEMENT_3D('',#12216,#9868,#9869);
#8670=AXIS2_PLACEMENT_3D('',#12218,#9870,#9871);
#8671=AXIS2_PLACEMENT_3D('',#12219,#9872,#9873);
#8672=AXIS2_PLACEMENT_3D('',#12220,#9874,#9875);
#8673=AXIS2_PLACEMENT_3D('',#12244,#9876,#9877);
#8674=AXIS2_PLACEMENT_3D('',#12245,#9878,#9879);
#8675=AXIS2_PLACEMENT_3D('',#12247,#9880,#9881);
#8676=AXIS2_PLACEMENT_3D('',#12250,#9883,#9884);
#8677=AXIS2_PLACEMENT_3D('',#12274,#9885,#9886);
#8678=AXIS2_PLACEMENT_3D('',#12275,#9887,#9888);
#8679=AXIS2_PLACEMENT_3D('',#12276,#9889,#9890);
#8680=AXIS2_PLACEMENT_3D('',#12277,#9891,#9892);
#8681=AXIS2_PLACEMENT_3D('',#12278,#9893,#9894);
#8682=AXIS2_PLACEMENT_3D('',#12279,#9895,#9896);
#8683=AXIS2_PLACEMENT_3D('',#12280,#9897,#9898);
#9789=DIRECTION('axis',(0.,0.,1.));
#9790=DIRECTION('refdir',(1.,0.,0.));
#9791=DIRECTION('center_axis',(0.,0.,1.));
#9792=DIRECTION('ref_axis',(1.,0.,0.));
#9793=DIRECTION('center_axis',(0.,-1.,0.));
#9794=DIRECTION('ref_axis',(0.,0.,-1.));
#9795=DIRECTION('center_axis',(0.,-1.,0.));
#9796=DIRECTION('ref_axis',(0.,0.,-1.));
#9797=DIRECTION('center_axis',(0.,1.,0.));
#9798=DIRECTION('ref_axis',(1.,0.,0.));
#9799=DIRECTION('center_axis',(0.,1.,0.));
#9800=DIRECTION('ref_axis',(1.,0.,0.));
#9801=DIRECTION('center_axis',(0.,1.,0.));
#9802=DIRECTION('ref_axis',(1.,0.,0.));
#9803=DIRECTION('center_axis',(0.,1.,0.));
#9804=DIRECTION('ref_axis',(1.,0.,0.));
#9805=DIRECTION('',(0.,-1.,0.));
#9806=DIRECTION('center_axis',(0.,-1.,0.));
#9807=DIRECTION('ref_axis',(1.,0.,0.));
#9808=DIRECTION('center_axis',(0.,1.,0.));
#9809=DIRECTION('ref_axis',(1.,0.,0.));
#9810=DIRECTION('center_axis',(0.,1.,0.));
#9811=DIRECTION('ref_axis',(1.,0.,0.));
#9812=DIRECTION('center_axis',(0.,1.,0.));
#9813=DIRECTION('ref_axis',(1.,0.,0.));
#9814=DIRECTION('center_axis',(0.,1.,0.));
#9815=DIRECTION('ref_axis',(1.,0.,0.));
#9816=DIRECTION('center_axis',(0.,1.,0.));
#9817=DIRECTION('ref_axis',(1.,0.,0.));
#9818=DIRECTION('center_axis',(0.,1.,0.));
#9819=DIRECTION('ref_axis',(1.,0.,0.));
#9820=DIRECTION('center_axis',(0.,-1.,0.));
#9821=DIRECTION('ref_axis',(1.,0.,0.));
#9822=DIRECTION('center_axis',(0.,-1.,0.));
#9823=DIRECTION('ref_axis',(0.,0.,-1.));
#9824=DIRECTION('center_axis',(6.12323399573677E-17,0.,1.));
#9825=DIRECTION('ref_axis',(1.,0.,0.));
#9826=DIRECTION('center_axis',(0.,-1.,0.));
#9827=DIRECTION('ref_axis',(0.,0.,-1.));
#9828=DIRECTION('center_axis',(0.,1.,0.));
#9829=DIRECTION('ref_axis',(1.,0.,0.));
#9830=DIRECTION('center_axis',(0.,-1.,0.));
#9831=DIRECTION('ref_axis',(1.,0.,0.));
#9832=DIRECTION('center_axis',(0.,-1.,0.));
#9833=DIRECTION('ref_axis',(0.,0.,-1.));
#9834=DIRECTION('center_axis',(0.,0.,1.));
#9835=DIRECTION('ref_axis',(1.,0.,0.));
#9836=DIRECTION('center_axis',(0.,-1.,0.));
#9837=DIRECTION('ref_axis',(0.,0.,-1.));
#9838=DIRECTION('center_axis',(0.,1.,0.));
#9839=DIRECTION('ref_axis',(1.,0.,0.));
#9840=DIRECTION('center_axis',(0.,-1.,0.));
#9841=DIRECTION('ref_axis',(1.,0.,0.));
#9842=DIRECTION('center_axis',(0.,-1.,0.));
#9843=DIRECTION('ref_axis',(0.,0.,-1.));
#9844=DIRECTION('center_axis',(0.,0.,1.));
#9845=DIRECTION('ref_axis',(1.,0.,0.));
#9846=DIRECTION('center_axis',(0.,-1.,0.));
#9847=DIRECTION('ref_axis',(0.,0.,-1.));
#9848=DIRECTION('center_axis',(0.,1.,0.));
#9849=DIRECTION('ref_axis',(1.,0.,0.));
#9850=DIRECTION('center_axis',(0.,-1.,0.));
#9851=DIRECTION('ref_axis',(1.,0.,0.));
#9852=DIRECTION('center_axis',(0.,-1.,0.));
#9853=DIRECTION('ref_axis',(0.,0.,-1.));
#9854=DIRECTION('center_axis',(0.,0.,1.));
#9855=DIRECTION('ref_axis',(1.,0.,0.));
#9856=DIRECTION('center_axis',(0.,-1.,0.));
#9857=DIRECTION('ref_axis',(0.,0.,-1.));
#9858=DIRECTION('center_axis',(0.,1.,0.));
#9859=DIRECTION('ref_axis',(1.,0.,0.));
#9860=DIRECTION('center_axis',(0.,-1.,0.));
#9861=DIRECTION('ref_axis',(1.,0.,0.));
#9862=DIRECTION('center_axis',(0.,-1.,0.));
#9863=DIRECTION('ref_axis',(0.,0.,-1.));
#9864=DIRECTION('center_axis',(6.12323399573676E-17,0.,1.));
#9865=DIRECTION('ref_axis',(1.,0.,0.));
#9866=DIRECTION('center_axis',(0.,-1.,0.));
#9867=DIRECTION('ref_axis',(0.,0.,-1.));
#9868=DIRECTION('center_axis',(0.,1.,0.));
#9869=DIRECTION('ref_axis',(1.,0.,0.));
#9870=DIRECTION('center_axis',(0.,-1.,0.));
#9871=DIRECTION('ref_axis',(1.,0.,0.));
#9872=DIRECTION('center_axis',(0.,-1.,0.));
#9873=DIRECTION('ref_axis',(0.,0.,-1.));
#9874=DIRECTION('center_axis',(0.,0.,1.));
#9875=DIRECTION('ref_axis',(1.,0.,0.));
#9876=DIRECTION('center_axis',(0.,-1.,0.));
#9877=DIRECTION('ref_axis',(0.,0.,-1.));
#9878=DIRECTION('center_axis',(0.,1.,0.));
#9879=DIRECTION('ref_axis',(1.,0.,0.));
#9880=DIRECTION('center_axis',(0.,1.,0.));
#9881=DIRECTION('ref_axis',(1.,0.,0.));
#9882=DIRECTION('',(0.,1.,0.));
#9883=DIRECTION('center_axis',(0.,-1.,0.));
#9884=DIRECTION('ref_axis',(1.,0.,0.));
#9885=DIRECTION('center_axis',(0.,-1.,0.));
#9886=DIRECTION('ref_axis',(1.,0.,0.));
#9887=DIRECTION('center_axis',(0.,1.,0.));
#9888=DIRECTION('ref_axis',(1.,0.,0.));
#9889=DIRECTION('center_axis',(0.,-1.,0.));
#9890=DIRECTION('ref_axis',(0.,0.,-1.));
#9891=DIRECTION('center_axis',(0.,0.,1.));
#9892=DIRECTION('ref_axis',(1.,0.,0.));
#9893=DIRECTION('center_axis',(0.,-1.,0.));
#9894=DIRECTION('ref_axis',(0.,0.,-1.));
#9895=DIRECTION('center_axis',(0.,-1.,0.));
#9896=DIRECTION('ref_axis',(-1.,0.,0.));
#9897=DIRECTION('center_axis',(0.,1.,0.));
#9898=DIRECTION('ref_axis',(1.,0.,0.));
#11833=CARTESIAN_POINT('',(0.,0.,0.));
#11834=CARTESIAN_POINT('Origin',(1.18440385848747,0.,1.18440385848747));
#11835=CARTESIAN_POINT('',(0.846804978391753,-0.07938,1.40825612658882));
#11836=CARTESIAN_POINT('',(1.40825612658882,-0.07938,0.846804978391754));
#11837=CARTESIAN_POINT('Ctrl Pts',(0.846804978391752,-0.0793800000000001,
1.40825612658882));
#11838=CARTESIAN_POINT('Ctrl Pts',(0.854205272175554,-0.123401821157026,
1.40380622184538));
#11839=CARTESIAN_POINT('Ctrl Pts',(0.867957148219441,-0.166543350814306,
1.39550172959303));
#11840=CARTESIAN_POINT('Ctrl Pts',(0.902193646979982,-0.237231147975234,
1.3735491215176));
#11841=CARTESIAN_POINT('Ctrl Pts',(0.920778333482564,-0.266264900654909,
1.36127834356734));
#11842=CARTESIAN_POINT('Ctrl Pts',(0.962485392528369,-0.317195968905306,
1.33211611256184));
#11843=CARTESIAN_POINT('Ctrl Pts',(0.985600426557816,-0.33909093068465,
1.31521005565926));
#11844=CARTESIAN_POINT('Ctrl Pts',(1.03253285680459,-0.373586846396559,
1.27866649102984));
#11845=CARTESIAN_POINT('Ctrl Pts',(1.05871835910697,-0.388086240756494,
1.25722555095714));
#11846=CARTESIAN_POINT('Ctrl Pts',(1.11153475808518,-0.407068917407805,
1.2107812086231));
#11847=CARTESIAN_POINT('Ctrl Pts',(1.13814686046673,-0.411552957311693,
1.18575674747573));
#11848=CARTESIAN_POINT('Ctrl Pts',(1.18575674747573,-0.411552957311693,
1.13814686046673));
#11849=CARTESIAN_POINT('Ctrl Pts',(1.2107812086231,-0.407068917407805,1.11153475808518));
#11850=CARTESIAN_POINT('Ctrl Pts',(1.25722555095713,-0.388086240756494,
1.05871835910697));
#11851=CARTESIAN_POINT('Ctrl Pts',(1.27866649102984,-0.373586846396559,
1.03253285680459));
#11852=CARTESIAN_POINT('Ctrl Pts',(1.31521005565926,-0.33909093068465,0.985600426557816));
#11853=CARTESIAN_POINT('Ctrl Pts',(1.33211611256184,-0.317195968905306,
0.962485392528369));
#11854=CARTESIAN_POINT('Ctrl Pts',(1.36127834356734,-0.266264900654909,
0.920778333482565));
#11855=CARTESIAN_POINT('Ctrl Pts',(1.3735491215176,-0.237231147975234,0.902193646979983));
#11856=CARTESIAN_POINT('Ctrl Pts',(1.39550172959303,-0.166543350814306,
0.867957148219442));
#11857=CARTESIAN_POINT('Ctrl Pts',(1.40380622184538,-0.123401821157026,
0.854205272175555));
#11858=CARTESIAN_POINT('Ctrl Pts',(1.40825612658882,-0.0793800000000001,
0.846804978391753));
#11859=CARTESIAN_POINT('',(0.886256117232623,-0.07938,1.45861320581289));
#11860=CARTESIAN_POINT('Origin',(1.18440385848747,-0.07938,1.18440385848747));
#11861=CARTESIAN_POINT('',(1.45861320581289,-0.07938,0.886256117232624));
#11862=CARTESIAN_POINT('Ctrl Pts',(1.45861320581289,-0.0793800000000001,
0.886256117232623));
#11863=CARTESIAN_POINT('Ctrl Pts',(1.45630208793976,-0.101649918886749,
0.890059788636852));
#11864=CARTESIAN_POINT('Ctrl Pts',(1.45296717977858,-0.123823518623746,
0.895520212222107));
#11865=CARTESIAN_POINT('Ctrl Pts',(1.43904931717599,-0.192480977588836,
0.917859913453975));
#11866=CARTESIAN_POINT('Ctrl Pts',(1.4243271592157,-0.236152929235938,0.940896403863072));
#11867=CARTESIAN_POINT('Ctrl Pts',(1.39055359345152,-0.303141259068212,
0.990027513266106));
#11868=CARTESIAN_POINT('Ctrl Pts',(1.36743459453896,-0.335108247315849,
1.02199477007745));
#11869=CARTESIAN_POINT('Ctrl Pts',(1.32643091652006,-0.373243761060364,
1.07446535104584));
#11870=CARTESIAN_POINT('Ctrl Pts',(1.30441816675528,-0.387888272594439,
1.10126842659597));
#11871=CARTESIAN_POINT('Ctrl Pts',(1.25681160160691,-0.407041111792943,
1.15530234155453));
#11872=CARTESIAN_POINT('Ctrl Pts',(1.23119764287622,-0.411552957311693,
1.18251418313119));
#11873=CARTESIAN_POINT('Ctrl Pts',(1.18251418313119,-0.411552957311693,
1.23119764287622));
#11874=CARTESIAN_POINT('Ctrl Pts',(1.15530234155453,-0.407041111792943,
1.25681160160691));
#11875=CARTESIAN_POINT('Ctrl Pts',(1.10126842659597,-0.387888272594439,
1.30441816675528));
#11876=CARTESIAN_POINT('Ctrl Pts',(1.07446535104584,-0.373243761060364,
1.32643091652006));
#11877=CARTESIAN_POINT('Ctrl Pts',(1.02199477007745,-0.335108247315848,
1.36743459453896));
#11878=CARTESIAN_POINT('Ctrl Pts',(0.990027513266105,-0.303141259068211,
1.39055359345152));
#11879=CARTESIAN_POINT('Ctrl Pts',(0.940896403863071,-0.236152929235937,
1.42432715921571));
#11880=CARTESIAN_POINT('Ctrl Pts',(0.917859913453974,-0.192480977588835,
1.43904931717599));
#11881=CARTESIAN_POINT('Ctrl Pts',(0.895520212222106,-0.123823518623745,
1.45296717977858));
#11882=CARTESIAN_POINT('Ctrl Pts',(0.890059788636851,-0.101649918886749,
1.45630208793976));
#11883=CARTESIAN_POINT('Ctrl Pts',(0.886256117232622,-0.0793800000000001,
1.45861320581289));
#11884=CARTESIAN_POINT('Origin',(1.18440385848747,-0.07938,1.18440385848747));
#11885=CARTESIAN_POINT('Origin',(0.,-0.27783,0.));
#11886=CARTESIAN_POINT('',(0.404717578595295,-0.07938,1.65807299932179));
#11887=CARTESIAN_POINT('Origin',(0.,-0.07938,0.));
#11888=CARTESIAN_POINT('',(-0.404717578595296,-0.07938,1.65807299932179));
#11889=CARTESIAN_POINT('Ctrl Pts',(0.404717578595296,-0.0793800000000001,
1.65807299932179));
#11890=CARTESIAN_POINT('Ctrl Pts',(0.400393769631747,-0.101649918886749,
1.65912839404491));
#11891=CARTESIAN_POINT('Ctrl Pts',(0.394174530911058,-0.123823518623745,
1.66063136041479));
#11892=CARTESIAN_POINT('Ctrl Pts',(0.368536561654407,-0.192480977588835,
1.66658649961961));
#11893=CARTESIAN_POINT('Ctrl Pts',(0.341837165343982,-0.236152929235937,
1.67246562047521));
#11894=CARTESIAN_POINT('Ctrl Pts',(0.283214707341173,-0.303141259068211,
1.68332504372461));
#11895=CARTESIAN_POINT('Ctrl Pts',(0.244262842368623,-0.335108247315849,
1.68958170688653));
#11896=CARTESIAN_POINT('Ctrl Pts',(0.178166559972324,-0.373243761060364,
1.69769003172132));
#11897=CARTESIAN_POINT('Ctrl Pts',(0.143648558862931,-0.387888272594439,
1.70107730356824));
#11898=CARTESIAN_POINT('Ctrl Pts',(0.0717778861362652,-0.407041111792943,
1.70562212620408));
#11899=CARTESIAN_POINT('Ctrl Pts',(0.0344244045173309,-0.411552957311693,
1.706752));
#11900=CARTESIAN_POINT('Ctrl Pts',(-0.0344244045173315,-0.411552957311693,
1.706752));
#11901=CARTESIAN_POINT('Ctrl Pts',(-0.0717778861362658,-0.407041111792943,
1.70562212620408));
#11902=CARTESIAN_POINT('Ctrl Pts',(-0.143648558862932,-0.387888272594439,
1.70107730356824));
#11903=CARTESIAN_POINT('Ctrl Pts',(-0.178166559972325,-0.373243761060364,
1.69769003172132));
#11904=CARTESIAN_POINT('Ctrl Pts',(-0.244262842368624,-0.335108247315849,
1.68958170688653));
#11905=CARTESIAN_POINT('Ctrl Pts',(-0.283214707341173,-0.303141259068212,
1.68332504372461));
#11906=CARTESIAN_POINT('Ctrl Pts',(-0.341837165343982,-0.236152929235937,
1.67246562047521));
#11907=CARTESIAN_POINT('Ctrl Pts',(-0.368536561654408,-0.192480977588835,
1.66658649961961));
#11908=CARTESIAN_POINT('Ctrl Pts',(-0.394174530911059,-0.123823518623745,
1.66063136041479));
#11909=CARTESIAN_POINT('Ctrl Pts',(-0.400393769631748,-0.101649918886749,
1.65912839404491));
#11910=CARTESIAN_POINT('Ctrl Pts',(-0.404717578595297,-0.0793800000000001,
1.65807299932179));
#11911=CARTESIAN_POINT('',(-0.886256117232624,-0.07938,1.45861320581289));
#11912=CARTESIAN_POINT('Origin',(0.,-0.07938,0.));
#11913=CARTESIAN_POINT('',(-1.45861320581289,-0.07938,0.886256117232623));
#11914=CARTESIAN_POINT('Ctrl Pts',(-0.886256117232623,-0.0793800000000001,
1.45861320581289));
#11915=CARTESIAN_POINT('Ctrl Pts',(-0.890059788636852,-0.101649918886749,
1.45630208793976));
#11916=CARTESIAN_POINT('Ctrl Pts',(-0.895520212222106,-0.123823518623745,
1.45296717977858));
#11917=CARTESIAN_POINT('Ctrl Pts',(-0.917859913453974,-0.192480977588835,
1.43904931717599));
#11918=CARTESIAN_POINT('Ctrl Pts',(-0.940896403863071,-0.236152929235937,
1.4243271592157));
#11919=CARTESIAN_POINT('Ctrl Pts',(-0.990027513266105,-0.303141259068211,
1.39055359345152));
#11920=CARTESIAN_POINT('Ctrl Pts',(-1.02199477007745,-0.335108247315848,
1.36743459453896));
#11921=CARTESIAN_POINT('Ctrl Pts',(-1.07446535104584,-0.373243761060364,
1.32643091652006));
#11922=CARTESIAN_POINT('Ctrl Pts',(-1.10126842659597,-0.387888272594439,
1.30441816675528));
#11923=CARTESIAN_POINT('Ctrl Pts',(-1.15530234155453,-0.407041111792943,
1.25681160160691));
#11924=CARTESIAN_POINT('Ctrl Pts',(-1.18251418313119,-0.411552957311693,
1.23119764287622));
#11925=CARTESIAN_POINT('Ctrl Pts',(-1.23119764287622,-0.411552957311693,
1.18251418313119));
#11926=CARTESIAN_POINT('Ctrl Pts',(-1.25681160160691,-0.407041111792943,
1.15530234155453));
#11927=CARTESIAN_POINT('Ctrl Pts',(-1.30441816675528,-0.387888272594439,
1.10126842659597));
#11928=CARTESIAN_POINT('Ctrl Pts',(-1.32643091652006,-0.373243761060365,
1.07446535104584));
#11929=CARTESIAN_POINT('Ctrl Pts',(-1.36743459453896,-0.335108247315849,
1.02199477007745));
#11930=CARTESIAN_POINT('Ctrl Pts',(-1.39055359345152,-0.303141259068212,
0.990027513266106));
#11931=CARTESIAN_POINT('Ctrl Pts',(-1.4243271592157,-0.236152929235938,
0.940896403863071));
#11932=CARTESIAN_POINT('Ctrl Pts',(-1.43904931717599,-0.192480977588836,
0.917859913453974));
#11933=CARTESIAN_POINT('Ctrl Pts',(-1.45296717977858,-0.123823518623746,
0.895520212222106));
#11934=CARTESIAN_POINT('Ctrl Pts',(-1.45630208793976,-0.101649918886749,
0.890059788636852));
#11935=CARTESIAN_POINT('Ctrl Pts',(-1.45861320581289,-0.0793800000000001,
0.886256117232623));
#11936=CARTESIAN_POINT('',(-1.65807299932179,-0.07938,0.404717578595295));
#11937=CARTESIAN_POINT('Origin',(0.,-0.07938,0.));
#11938=CARTESIAN_POINT('',(-1.706752,-0.411552957311693,2.08591827245526E-16));
#11939=CARTESIAN_POINT('Ctrl Pts',(-1.65807299932179,-0.0793800000000001,
0.404717578595296));
#11940=CARTESIAN_POINT('Ctrl Pts',(-1.65912839404491,-0.101649918886749,
0.400393769631747));
#11941=CARTESIAN_POINT('Ctrl Pts',(-1.66063136041479,-0.123823518623745,
0.394174530911058));
#11942=CARTESIAN_POINT('Ctrl Pts',(-1.66658649961961,-0.192480977588835,
0.368536561654407));
#11943=CARTESIAN_POINT('Ctrl Pts',(-1.67246562047521,-0.236152929235937,
0.341837165343982));
#11944=CARTESIAN_POINT('Ctrl Pts',(-1.68332504372461,-0.303141259068211,
0.283214707341173));
#11945=CARTESIAN_POINT('Ctrl Pts',(-1.68958170688653,-0.335108247315848,
0.244262842368623));
#11946=CARTESIAN_POINT('Ctrl Pts',(-1.69769003172132,-0.373243761060364,
0.178166559972324));
#11947=CARTESIAN_POINT('Ctrl Pts',(-1.70107730356824,-0.387888272594439,
0.143648558862931));
#11948=CARTESIAN_POINT('Ctrl Pts',(-1.70562212620408,-0.407041111792943,
0.0717778861362656));
#11949=CARTESIAN_POINT('Ctrl Pts',(-1.706752,-0.411552957311693,0.0344244045173313));
#11950=CARTESIAN_POINT('Ctrl Pts',(-1.706752,-0.411552957311693,2.08166817117217E-16));
#11951=CARTESIAN_POINT('',(-1.706752,-0.47628,2.09016837373834E-16));
#11952=CARTESIAN_POINT('',(-1.706752,-0.27783,2.09016837373834E-16));
#11953=CARTESIAN_POINT('Origin',(0.,-0.47628,0.));
#11954=CARTESIAN_POINT('',(-1.65807299932179,-0.07938,-0.404717578595296));
#11955=CARTESIAN_POINT('Ctrl Pts',(-1.706752,-0.411552957311693,2.0122792321331E-16));
#11956=CARTESIAN_POINT('Ctrl Pts',(-1.706752,-0.411552957311693,-0.0344244045173309));
#11957=CARTESIAN_POINT('Ctrl Pts',(-1.70562212620408,-0.407041111792943,
-0.0717778861362652));
#11958=CARTESIAN_POINT('Ctrl Pts',(-1.70107730356824,-0.387888272594439,
-0.143648558862931));
#11959=CARTESIAN_POINT('Ctrl Pts',(-1.69769003172132,-0.373243761060365,
-0.178166559972324));
#11960=CARTESIAN_POINT('Ctrl Pts',(-1.68958170688653,-0.335108247315849,
-0.244262842368623));
#11961=CARTESIAN_POINT('Ctrl Pts',(-1.68332504372461,-0.303141259068212,
-0.283214707341173));
#11962=CARTESIAN_POINT('Ctrl Pts',(-1.67246562047521,-0.236152929235938,
-0.341837165343982));
#11963=CARTESIAN_POINT('Ctrl Pts',(-1.66658649961961,-0.192480977588836,
-0.368536561654407));
#11964=CARTESIAN_POINT('Ctrl Pts',(-1.66063136041479,-0.123823518623745,
-0.394174530911059));
#11965=CARTESIAN_POINT('Ctrl Pts',(-1.65912839404491,-0.101649918886749,
-0.400393769631748));
#11966=CARTESIAN_POINT('Ctrl Pts',(-1.65807299932179,-0.0793800000000001,
-0.404717578595296));
#11967=CARTESIAN_POINT('',(-1.45861320581289,-0.07938,-0.886256117232623));
#11968=CARTESIAN_POINT('Origin',(0.,-0.07938,0.));
#11969=CARTESIAN_POINT('',(-0.886256117232623,-0.07938,-1.45861320581289));
#11970=CARTESIAN_POINT('Ctrl Pts',(-1.45861320581289,-0.0793800000000001,
-0.886256117232623));
#11971=CARTESIAN_POINT('Ctrl Pts',(-1.45630208793976,-0.101649918886749,
-0.890059788636852));
#11972=CARTESIAN_POINT('Ctrl Pts',(-1.45296717977858,-0.123823518623745,
-0.895520212222106));
#11973=CARTESIAN_POINT('Ctrl Pts',(-1.43904931717599,-0.192480977588835,
-0.917859913453974));
#11974=CARTESIAN_POINT('Ctrl Pts',(-1.4243271592157,-0.236152929235937,
-0.940896403863072));
#11975=CARTESIAN_POINT('Ctrl Pts',(-1.39055359345152,-0.303141259068212,
-0.990027513266106));
#11976=CARTESIAN_POINT('Ctrl Pts',(-1.36743459453896,-0.335108247315849,
-1.02199477007745));
#11977=CARTESIAN_POINT('Ctrl Pts',(-1.32643091652006,-0.373243761060364,
-1.07446535104584));
#11978=CARTESIAN_POINT('Ctrl Pts',(-1.30441816675528,-0.387888272594439,
-1.10126842659597));
#11979=CARTESIAN_POINT('Ctrl Pts',(-1.25681160160691,-0.407041111792943,
-1.15530234155453));
#11980=CARTESIAN_POINT('Ctrl Pts',(-1.23119764287622,-0.411552957311693,
-1.18251418313119));
#11981=CARTESIAN_POINT('Ctrl Pts',(-1.18251418313119,-0.411552957311693,
-1.23119764287622));
#11982=CARTESIAN_POINT('Ctrl Pts',(-1.15530234155453,-0.407041111792943,
-1.25681160160691));
#11983=CARTESIAN_POINT('Ctrl Pts',(-1.10126842659597,-0.387888272594439,
-1.30441816675528));
#11984=CARTESIAN_POINT('Ctrl Pts',(-1.07446535104584,-0.373243761060364,
-1.32643091652006));
#11985=CARTESIAN_POINT('Ctrl Pts',(-1.02199477007745,-0.335108247315848,
-1.36743459453896));
#11986=CARTESIAN_POINT('Ctrl Pts',(-0.990027513266105,-0.303141259068211,
-1.39055359345152));
#11987=CARTESIAN_POINT('Ctrl Pts',(-0.940896403863071,-0.236152929235936,
-1.42432715921571));
#11988=CARTESIAN_POINT('Ctrl Pts',(-0.917859913453974,-0.192480977588835,
-1.43904931717599));
#11989=CARTESIAN_POINT('Ctrl Pts',(-0.895520212222106,-0.123823518623745,
-1.45296717977858));
#11990=CARTESIAN_POINT('Ctrl Pts',(-0.890059788636851,-0.101649918886749,
-1.45630208793976));
#11991=CARTESIAN_POINT('Ctrl Pts',(-0.886256117232623,-0.0793800000000001,
-1.45861320581289));
#11992=CARTESIAN_POINT('',(-0.404717578595295,-0.07938,-1.65807299932179));
#11993=CARTESIAN_POINT('Origin',(0.,-0.07938,0.));
#11994=CARTESIAN_POINT('',(0.404717578595296,-0.07938,-1.65807299932179));
#11995=CARTESIAN_POINT('Ctrl Pts',(-0.404717578595296,-0.0793800000000001,
-1.65807299932179));
#11996=CARTESIAN_POINT('Ctrl Pts',(-0.400393769631747,-0.101649918886749,
-1.65912839404491));
#11997=CARTESIAN_POINT('Ctrl Pts',(-0.394174530911058,-0.123823518623746,
-1.66063136041479));
#11998=CARTESIAN_POINT('Ctrl Pts',(-0.368536561654407,-0.192480977588836,
-1.66658649961961));
#11999=CARTESIAN_POINT('Ctrl Pts',(-0.341837165343982,-0.236152929235938,
-1.67246562047521));
#12000=CARTESIAN_POINT('Ctrl Pts',(-0.283214707341173,-0.303141259068212,
-1.68332504372461));
#12001=CARTESIAN_POINT('Ctrl Pts',(-0.244262842368623,-0.335108247315849,
-1.68958170688653));
#12002=CARTESIAN_POINT('Ctrl Pts',(-0.178166559972324,-0.373243761060364,
-1.69769003172132));
#12003=CARTESIAN_POINT('Ctrl Pts',(-0.143648558862931,-0.387888272594439,
-1.70107730356824));
#12004=CARTESIAN_POINT('Ctrl Pts',(-0.0717778861362653,-0.407041111792943,
-1.70562212620408));
#12005=CARTESIAN_POINT('Ctrl Pts',(-0.034424404517331,-0.411552957311693,
-1.706752));
#12006=CARTESIAN_POINT('Ctrl Pts',(0.0344244045173312,-0.411552957311693,
-1.706752));
#12007=CARTESIAN_POINT('Ctrl Pts',(0.0717778861362655,-0.407041111792943,
-1.70562212620408));
#12008=CARTESIAN_POINT('Ctrl Pts',(0.143648558862931,-0.387888272594439,
-1.70107730356824));
#12009=CARTESIAN_POINT('Ctrl Pts',(0.178166559972324,-0.373243761060364,
-1.69769003172132));
#12010=CARTESIAN_POINT('Ctrl Pts',(0.244262842368623,-0.335108247315849,
-1.68958170688653));
#12011=CARTESIAN_POINT('Ctrl Pts',(0.283214707341173,-0.303141259068212,
-1.68332504372461));
#12012=CARTESIAN_POINT('Ctrl Pts',(0.341837165343982,-0.236152929235937,
-1.67246562047521));
#12013=CARTESIAN_POINT('Ctrl Pts',(0.368536561654407,-0.192480977588835,
-1.66658649961961));
#12014=CARTESIAN_POINT('Ctrl Pts',(0.394174530911059,-0.123823518623745,
-1.66063136041479));
#12015=CARTESIAN_POINT('Ctrl Pts',(0.400393769631748,-0.101649918886749,
-1.65912839404491));
#12016=CARTESIAN_POINT('Ctrl Pts',(0.404717578595296,-0.0793800000000001,
-1.65807299932179));
#12017=CARTESIAN_POINT('',(0.886256117232623,-0.07938,-1.45861320581289));
#12018=CARTESIAN_POINT('Origin',(0.,-0.07938,0.));
#12019=CARTESIAN_POINT('',(1.45861320581289,-0.07938,-0.886256117232623));
#12020=CARTESIAN_POINT('Ctrl Pts',(0.886256117232623,-0.0793800000000001,
-1.45861320581289));
#12021=CARTESIAN_POINT('Ctrl Pts',(0.890059788636852,-0.101649918886749,
-1.45630208793976));
#12022=CARTESIAN_POINT('Ctrl Pts',(0.895520212222106,-0.123823518623745,
-1.45296717977858));
#12023=CARTESIAN_POINT('Ctrl Pts',(0.917859913453974,-0.192480977588835,
-1.43904931717599));
#12024=CARTESIAN_POINT('Ctrl Pts',(0.940896403863072,-0.236152929235937,
-1.4243271592157));
#12025=CARTESIAN_POINT('Ctrl Pts',(0.990027513266106,-0.303141259068211,
-1.39055359345152));
#12026=CARTESIAN_POINT('Ctrl Pts',(1.02199477007745,-0.335108247315849,
-1.36743459453896));
#12027=CARTESIAN_POINT('Ctrl Pts',(1.07446535104584,-0.373243761060364,
-1.32643091652006));
#12028=CARTESIAN_POINT('Ctrl Pts',(1.10126842659597,-0.387888272594439,
-1.30441816675528));
#12029=CARTESIAN_POINT('Ctrl Pts',(1.15530234155453,-0.407041111792943,
-1.25681160160691));
#12030=CARTESIAN_POINT('Ctrl Pts',(1.18251418313119,-0.411552957311693,
-1.23119764287622));
#12031=CARTESIAN_POINT('Ctrl Pts',(1.23119764287622,-0.411552957311693,
-1.18251418313119));
#12032=CARTESIAN_POINT('Ctrl Pts',(1.25681160160691,-0.407041111792943,
-1.15530234155453));
#12033=CARTESIAN_POINT('Ctrl Pts',(1.30441816675528,-0.387888272594439,
-1.10126842659597));
#12034=CARTESIAN_POINT('Ctrl Pts',(1.32643091652006,-0.373243761060364,
-1.07446535104584));
#12035=CARTESIAN_POINT('Ctrl Pts',(1.36743459453896,-0.335108247315849,
-1.02199477007745));
#12036=CARTESIAN_POINT('Ctrl Pts',(1.39055359345152,-0.303141259068212,
-0.990027513266105));
#12037=CARTESIAN_POINT('Ctrl Pts',(1.4243271592157,-0.236152929235937,-0.940896403863071));
#12038=CARTESIAN_POINT('Ctrl Pts',(1.43904931717599,-0.192480977588835,
-0.917859913453974));
#12039=CARTESIAN_POINT('Ctrl Pts',(1.45296717977858,-0.123823518623745,
-0.895520212222106));
#12040=CARTESIAN_POINT('Ctrl Pts',(1.45630208793976,-0.101649918886749,
-0.890059788636852));
#12041=CARTESIAN_POINT('Ctrl Pts',(1.45861320581289,-0.0793800000000001,
-0.886256117232623));
#12042=CARTESIAN_POINT('',(1.65807299932179,-0.07938,-0.404717578595296));
#12043=CARTESIAN_POINT('Origin',(0.,-0.07938,0.));
#12044=CARTESIAN_POINT('',(1.65807299932179,-0.07938,0.404717578595296));
#12045=CARTESIAN_POINT('Ctrl Pts',(1.65807299932179,-0.0793800000000001,
-0.404717578595296));
#12046=CARTESIAN_POINT('Ctrl Pts',(1.65912839404491,-0.101649918886749,
-0.400393769631747));
#12047=CARTESIAN_POINT('Ctrl Pts',(1.66063136041479,-0.123823518623745,
-0.394174530911058));
#12048=CARTESIAN_POINT('Ctrl Pts',(1.66658649961961,-0.192480977588835,
-0.368536561654407));
#12049=CARTESIAN_POINT('Ctrl Pts',(1.67246562047521,-0.236152929235937,
-0.341837165343982));
#12050=CARTESIAN_POINT('Ctrl Pts',(1.68332504372461,-0.303141259068212,
-0.283214707341173));
#12051=CARTESIAN_POINT('Ctrl Pts',(1.68958170688653,-0.335108247315849,
-0.244262842368623));
#12052=CARTESIAN_POINT('Ctrl Pts',(1.69769003172132,-0.373243761060364,
-0.178166559972324));
#12053=CARTESIAN_POINT('Ctrl Pts',(1.70107730356824,-0.387888272594439,
-0.143648558862931));
#12054=CARTESIAN_POINT('Ctrl Pts',(1.70562212620408,-0.407041111792943,
-0.0717778861362655));
#12055=CARTESIAN_POINT('Ctrl Pts',(1.706752,-0.411552957311693,-0.0344244045173312));
#12056=CARTESIAN_POINT('Ctrl Pts',(1.706752,-0.411552957311693,0.0344244045173312));
#12057=CARTESIAN_POINT('Ctrl Pts',(1.70562212620408,-0.407041111792943,
0.0717778861362655));
#12058=CARTESIAN_POINT('Ctrl Pts',(1.70107730356824,-0.387888272594439,
0.143648558862931));
#12059=CARTESIAN_POINT('Ctrl Pts',(1.69769003172132,-0.373243761060364,
0.178166559972324));
#12060=CARTESIAN_POINT('Ctrl Pts',(1.68958170688653,-0.335108247315849,
0.244262842368623));
#12061=CARTESIAN_POINT('Ctrl Pts',(1.68332504372461,-0.303141259068212,
0.283214707341173));
#12062=CARTESIAN_POINT('Ctrl Pts',(1.67246562047521,-0.236152929235937,
0.341837165343982));
#12063=CARTESIAN_POINT('Ctrl Pts',(1.66658649961961,-0.192480977588835,
0.368536561654407));
#12064=CARTESIAN_POINT('Ctrl Pts',(1.66063136041479,-0.123823518623745,
0.394174530911058));
#12065=CARTESIAN_POINT('Ctrl Pts',(1.65912839404491,-0.101649918886749,
0.400393769631747));
#12066=CARTESIAN_POINT('Ctrl Pts',(1.65807299932179,-0.0793800000000001,
0.404717578595296));
#12067=CARTESIAN_POINT('Origin',(0.,-0.07938,0.));
#12068=CARTESIAN_POINT('Origin',(0.,-0.07938,0.));
#12069=CARTESIAN_POINT('',(0.397005914195118,-0.07938,1.59456899932179));
#12070=CARTESIAN_POINT('Origin',(0.,-0.07938,0.));
#12071=CARTESIAN_POINT('Origin',(-3.33066907387547E-16,-0.07938,1.675));
#12072=CARTESIAN_POINT('Origin',(-3.33066907387547E-16,0.,1.675));
#12073=CARTESIAN_POINT('',(-0.397005914195118,-0.07938,1.59456899932179));
#12074=CARTESIAN_POINT('Ctrl Pts',(-0.397005914195119,-0.0793800000000001,
1.59456899932179));
#12075=CARTESIAN_POINT('Ctrl Pts',(-0.3886265584581,-0.123401821157026,
1.59665523941937));
#12076=CARTESIAN_POINT('Ctrl Pts',(-0.373030350867485,-0.166543350814306,
1.60050712143809));
#12077=CARTESIAN_POINT('Ctrl Pts',(-0.333298652394954,-0.237231147975234,
1.60919314384089));
#12078=CARTESIAN_POINT('Ctrl Pts',(-0.311480544243687,-0.266264900654909,
1.61365775139403));
#12079=CARTESIAN_POINT('Ctrl Pts',(-0.261368388670537,-0.317195968905306,
1.62252828437015));
#12080=CARTESIAN_POINT('Ctrl Pts',(-0.233069203882014,-0.33909093068465,
1.62691869420078));
#12081=CARTESIAN_POINT('Ctrl Pts',(-0.174042761838764,-0.373586846396559,
1.63426473152765));
#12082=CARTESIAN_POINT('Ctrl Pts',(-0.14036578147155,-0.388086240756494,
1.63761964365402));
#12083=CARTESIAN_POINT('Ctrl Pts',(-0.0701778381840615,-0.407068917407805,
1.64212536811722));
#12084=CARTESIAN_POINT('Ctrl Pts',(-0.0336652739555918,-0.411552957311693,
1.643248));
#12085=CARTESIAN_POINT('Ctrl Pts',(0.0336652739555913,-0.411552957311693,
1.643248));
#12086=CARTESIAN_POINT('Ctrl Pts',(0.070177838184061,-0.407068917407805,
1.64212536811722));
#12087=CARTESIAN_POINT('Ctrl Pts',(0.140365781471549,-0.388086240756494,
1.63761964365402));
#12088=CARTESIAN_POINT('Ctrl Pts',(0.174042761838763,-0.373586846396559,
1.63426473152765));
#12089=CARTESIAN_POINT('Ctrl Pts',(0.233069203882014,-0.33909093068465,
1.62691869420078));
#12090=CARTESIAN_POINT('Ctrl Pts',(0.261368388670536,-0.317195968905306,
1.62252828437015));
#12091=CARTESIAN_POINT('Ctrl Pts',(0.311480544243686,-0.266264900654908,
1.61365775139403));
#12092=CARTESIAN_POINT('Ctrl Pts',(0.333298652394954,-0.237231147975234,
1.60919314384089));
#12093=CARTESIAN_POINT('Ctrl Pts',(0.373030350867484,-0.166543350814306,
1.60050712143809));
#12094=CARTESIAN_POINT('Ctrl Pts',(0.388626558458099,-0.123401821157026,
1.59665523941937));
#12095=CARTESIAN_POINT('Ctrl Pts',(0.397005914195118,-0.07938,1.59456899932179));
#12096=CARTESIAN_POINT('Origin',(-3.33066907387547E-16,-0.07938,1.675));
#12097=CARTESIAN_POINT('Origin',(0.,-0.07938,0.));
#12098=CARTESIAN_POINT('',(-0.846804978391754,-0.07938,1.40825612658882));
#12099=CARTESIAN_POINT('Origin',(0.,-0.07938,0.));
#12100=CARTESIAN_POINT('Origin',(-1.18440385848747,-0.07938,1.18440385848747));
#12101=CARTESIAN_POINT('Origin',(-1.18440385848747,0.,1.18440385848747));
#12102=CARTESIAN_POINT('',(-1.40825612658882,-0.07938,0.846804978391753));
#12103=CARTESIAN_POINT('Ctrl Pts',(-1.40825612658882,-0.0793800000000001,
0.846804978391753));
#12104=CARTESIAN_POINT('Ctrl Pts',(-1.40380622184538,-0.123401821157026,
0.854205272175555));
#12105=CARTESIAN_POINT('Ctrl Pts',(-1.39550172959303,-0.166543350814306,
0.867957148219442));
#12106=CARTESIAN_POINT('Ctrl Pts',(-1.3735491215176,-0.237231147975235,
0.902193646979983));
#12107=CARTESIAN_POINT('Ctrl Pts',(-1.36127834356734,-0.266264900654909,
0.920778333482565));
#12108=CARTESIAN_POINT('Ctrl Pts',(-1.33211611256184,-0.317195968905306,
0.962485392528369));
#12109=CARTESIAN_POINT('Ctrl Pts',(-1.31521005565926,-0.339090930684651,
0.985600426557816));
#12110=CARTESIAN_POINT('Ctrl Pts',(-1.27866649102984,-0.373586846396559,
1.03253285680459));
#12111=CARTESIAN_POINT('Ctrl Pts',(-1.25722555095714,-0.388086240756494,
1.05871835910697));
#12112=CARTESIAN_POINT('Ctrl Pts',(-1.2107812086231,-0.407068917407805,
1.11153475808518));
#12113=CARTESIAN_POINT('Ctrl Pts',(-1.18575674747573,-0.411552957311693,
1.13814686046673));
#12114=CARTESIAN_POINT('Ctrl Pts',(-1.13814686046673,-0.411552957311693,
1.18575674747573));
#12115=CARTESIAN_POINT('Ctrl Pts',(-1.11153475808518,-0.407068917407805,
1.2107812086231));
#12116=CARTESIAN_POINT('Ctrl Pts',(-1.05871835910697,-0.388086240756494,
1.25722555095714));
#12117=CARTESIAN_POINT('Ctrl Pts',(-1.03253285680459,-0.373586846396559,
1.27866649102984));
#12118=CARTESIAN_POINT('Ctrl Pts',(-0.985600426557816,-0.33909093068465,
1.31521005565926));
#12119=CARTESIAN_POINT('Ctrl Pts',(-0.962485392528369,-0.317195968905306,
1.33211611256184));
#12120=CARTESIAN_POINT('Ctrl Pts',(-0.920778333482565,-0.266264900654908,
1.36127834356734));
#12121=CARTESIAN_POINT('Ctrl Pts',(-0.902193646979983,-0.237231147975234,
1.3735491215176));
#12122=CARTESIAN_POINT('Ctrl Pts',(-0.867957148219442,-0.166543350814306,
1.39550172959303));
#12123=CARTESIAN_POINT('Ctrl Pts',(-0.854205272175555,-0.123401821157026,
1.40380622184538));
#12124=CARTESIAN_POINT('Ctrl Pts',(-0.846804978391753,-0.0793800000000001,
1.40825612658882));
#12125=CARTESIAN_POINT('Origin',(-1.18440385848747,-0.07938,1.18440385848747));
#12126=CARTESIAN_POINT('Origin',(0.,-0.07938,0.));
#12127=CARTESIAN_POINT('',(-1.59456899932179,-0.07938,0.397005914195118));
#12128=CARTESIAN_POINT('Origin',(0.,-0.07938,0.));
#12129=CARTESIAN_POINT('Origin',(-1.675,-0.07938,-2.22044604925031E-16));
#12130=CARTESIAN_POINT('Origin',(-1.675,0.,-2.22044604925031E-16));
#12131=CARTESIAN_POINT('',(-1.59456899932179,-0.07938,-0.397005914195118));
#12132=CARTESIAN_POINT('',(-1.643248,-0.411552957311693,3.47540551556327E-18));
#12133=CARTESIAN_POINT('Ctrl Pts',(-1.59456899932179,-0.0793800000000001,
-0.397005914195119));
#12134=CARTESIAN_POINT('Ctrl Pts',(-1.59665523941937,-0.123401821157026,
-0.388626558458099));
#12135=CARTESIAN_POINT('Ctrl Pts',(-1.60050712143809,-0.166543350814306,
-0.373030350867485));
#12136=CARTESIAN_POINT('Ctrl Pts',(-1.60919314384089,-0.237231147975234,
-0.333298652394954));
#12137=CARTESIAN_POINT('Ctrl Pts',(-1.61365775139403,-0.266264900654909,
-0.311480544243686));
#12138=CARTESIAN_POINT('Ctrl Pts',(-1.62252828437015,-0.317195968905306,
-0.261368388670537));
#12139=CARTESIAN_POINT('Ctrl Pts',(-1.62691869420078,-0.33909093068465,
-0.233069203882014));
#12140=CARTESIAN_POINT('Ctrl Pts',(-1.63426473152765,-0.373586846396559,
-0.174042761838764));
#12141=CARTESIAN_POINT('Ctrl Pts',(-1.63761964365402,-0.388086240756494,
-0.140365781471549));
#12142=CARTESIAN_POINT('Ctrl Pts',(-1.64212536811722,-0.407068917407805,
-0.0701778381840614));
#12143=CARTESIAN_POINT('Ctrl Pts',(-1.643248,-0.411552957311693,-0.0336652739555917));
#12144=CARTESIAN_POINT('Ctrl Pts',(-1.643248,-0.411552957311693,-2.0122792321331E-16));
#12145=CARTESIAN_POINT('Origin',(-1.675,-0.07938,-2.22044604925031E-16));
#12146=CARTESIAN_POINT('Ctrl Pts',(-1.643248,-0.411552957311693,-1.94289029309402E-16));
#12147=CARTESIAN_POINT('Ctrl Pts',(-1.643248,-0.411552957311693,0.0336652739555913));
#12148=CARTESIAN_POINT('Ctrl Pts',(-1.64212536811722,-0.407068917407805,
0.0701778381840609));
#12149=CARTESIAN_POINT('Ctrl Pts',(-1.63761964365402,-0.388086240756494,
0.140365781471549));
#12150=CARTESIAN_POINT('Ctrl Pts',(-1.63426473152765,-0.373586846396559,
0.174042761838763));
#12151=CARTESIAN_POINT('Ctrl Pts',(-1.62691869420078,-0.33909093068465,
0.233069203882014));
#12152=CARTESIAN_POINT('Ctrl Pts',(-1.62252828437015,-0.317195968905306,
0.261368388670536));
#12153=CARTESIAN_POINT('Ctrl Pts',(-1.61365775139403,-0.266264900654909,
0.311480544243686));
#12154=CARTESIAN_POINT('Ctrl Pts',(-1.60919314384089,-0.237231147975235,
0.333298652394954));
#12155=CARTESIAN_POINT('Ctrl Pts',(-1.60050712143809,-0.166543350814306,
0.373030350867484));
#12156=CARTESIAN_POINT('Ctrl Pts',(-1.59665523941937,-0.123401821157026,
0.388626558458099));
#12157=CARTESIAN_POINT('Ctrl Pts',(-1.59456899932179,-0.0793800000000001,
0.397005914195118));
#12158=CARTESIAN_POINT('Origin',(0.,-0.07938,0.));
#12159=CARTESIAN_POINT('',(-1.40825612658882,-0.07938,-0.846804978391753));
#12160=CARTESIAN_POINT('Origin',(0.,-0.07938,0.));
#12161=CARTESIAN_POINT('Origin',(-1.18440385848747,-0.07938,-1.18440385848747));
#12162=CARTESIAN_POINT('Origin',(-1.18440385848747,0.,-1.18440385848747));
#12163=CARTESIAN_POINT('',(-0.846804978391753,-0.07938,-1.40825612658882));
#12164=CARTESIAN_POINT('Ctrl Pts',(-0.846804978391753,-0.0793800000000001,
-1.40825612658882));
#12165=CARTESIAN_POINT('Ctrl Pts',(-0.854205272175555,-0.123401821157026,
-1.40380622184538));
#12166=CARTESIAN_POINT('Ctrl Pts',(-0.867957148219442,-0.166543350814306,
-1.39550172959303));
#12167=CARTESIAN_POINT('Ctrl Pts',(-0.902193646979982,-0.237231147975234,
-1.3735491215176));
#12168=CARTESIAN_POINT('Ctrl Pts',(-0.920778333482564,-0.266264900654908,
-1.36127834356734));
#12169=CARTESIAN_POINT('Ctrl Pts',(-0.962485392528368,-0.317195968905306,
-1.33211611256184));
#12170=CARTESIAN_POINT('Ctrl Pts',(-0.985600426557816,-0.33909093068465,
-1.31521005565926));
#12171=CARTESIAN_POINT('Ctrl Pts',(-1.03253285680459,-0.373586846396559,
-1.27866649102984));
#12172=CARTESIAN_POINT('Ctrl Pts',(-1.05871835910697,-0.388086240756494,
-1.25722555095714));
#12173=CARTESIAN_POINT('Ctrl Pts',(-1.11153475808518,-0.407068917407805,
-1.2107812086231));
#12174=CARTESIAN_POINT('Ctrl Pts',(-1.13814686046673,-0.411552957311693,
-1.18575674747573));
#12175=CARTESIAN_POINT('Ctrl Pts',(-1.18575674747573,-0.411552957311693,
-1.13814686046673));
#12176=CARTESIAN_POINT('Ctrl Pts',(-1.2107812086231,-0.407068917407805,
-1.11153475808518));
#12177=CARTESIAN_POINT('Ctrl Pts',(-1.25722555095714,-0.388086240756494,
-1.05871835910697));
#12178=CARTESIAN_POINT('Ctrl Pts',(-1.27866649102984,-0.373586846396559,
-1.03253285680459));
#12179=CARTESIAN_POINT('Ctrl Pts',(-1.31521005565926,-0.33909093068465,
-0.985600426557816));
#12180=CARTESIAN_POINT('Ctrl Pts',(-1.33211611256184,-0.317195968905306,
-0.962485392528369));
#12181=CARTESIAN_POINT('Ctrl Pts',(-1.36127834356734,-0.266264900654909,
-0.920778333482565));
#12182=CARTESIAN_POINT('Ctrl Pts',(-1.3735491215176,-0.237231147975234,
-0.902193646979983));
#12183=CARTESIAN_POINT('Ctrl Pts',(-1.39550172959303,-0.166543350814306,
-0.867957148219442));
#12184=CARTESIAN_POINT('Ctrl Pts',(-1.40380622184538,-0.123401821157026,
-0.854205272175555));
#12185=CARTESIAN_POINT('Ctrl Pts',(-1.40825612658882,-0.07938,-0.846804978391753));
#12186=CARTESIAN_POINT('Origin',(-1.18440385848747,-0.07938,-1.18440385848747));
#12187=CARTESIAN_POINT('Origin',(0.,-0.07938,0.));
#12188=CARTESIAN_POINT('',(-0.397005914195118,-0.07938,-1.59456899932179));
#12189=CARTESIAN_POINT('Origin',(0.,-0.07938,0.));
#12190=CARTESIAN_POINT('Origin',(1.11022302462516E-16,-0.07938,-1.675));
#12191=CARTESIAN_POINT('Origin',(1.11022302462516E-16,0.,-1.675));
#12192=CARTESIAN_POINT('',(0.397005914195118,-0.07938,-1.59456899932179));
#12193=CARTESIAN_POINT('Ctrl Pts',(0.397005914195119,-0.0793800000000001,
-1.59456899932179));
#12194=CARTESIAN_POINT('Ctrl Pts',(0.388626558458099,-0.123401821157026,
-1.59665523941937));
#12195=CARTESIAN_POINT('Ctrl Pts',(0.373030350867485,-0.166543350814306,
-1.60050712143809));
#12196=CARTESIAN_POINT('Ctrl Pts',(0.333298652394954,-0.237231147975234,
-1.60919314384089));
#12197=CARTESIAN_POINT('Ctrl Pts',(0.311480544243686,-0.266264900654909,
-1.61365775139403));
#12198=CARTESIAN_POINT('Ctrl Pts',(0.261368388670537,-0.317195968905306,
-1.62252828437015));
#12199=CARTESIAN_POINT('Ctrl Pts',(0.233069203882014,-0.33909093068465,
-1.62691869420078));
#12200=CARTESIAN_POINT('Ctrl Pts',(0.174042761838763,-0.373586846396559,
-1.63426473152765));
#12201=CARTESIAN_POINT('Ctrl Pts',(0.140365781471549,-0.388086240756494,
-1.63761964365402));
#12202=CARTESIAN_POINT('Ctrl Pts',(0.0701778381840612,-0.407068917407805,
-1.64212536811722));
#12203=CARTESIAN_POINT('Ctrl Pts',(0.0336652739555916,-0.411552957311693,
-1.643248));
#12204=CARTESIAN_POINT('Ctrl Pts',(-0.0336652739555915,-0.411552957311693,
-1.643248));
#12205=CARTESIAN_POINT('Ctrl Pts',(-0.0701778381840612,-0.407068917407805,
-1.64212536811722));
#12206=CARTESIAN_POINT('Ctrl Pts',(-0.140365781471549,-0.388086240756494,
-1.63761964365402));
#12207=CARTESIAN_POINT('Ctrl Pts',(-0.174042761838764,-0.373586846396559,
-1.63426473152765));
#12208=CARTESIAN_POINT('Ctrl Pts',(-0.233069203882014,-0.33909093068465,
-1.62691869420078));
#12209=CARTESIAN_POINT('Ctrl Pts',(-0.261368388670536,-0.317195968905306,
-1.62252828437015));
#12210=CARTESIAN_POINT('Ctrl Pts',(-0.311480544243686,-0.266264900654908,
-1.61365775139403));
#12211=CARTESIAN_POINT('Ctrl Pts',(-0.333298652394954,-0.237231147975234,
-1.60919314384089));
#12212=CARTESIAN_POINT('Ctrl Pts',(-0.373030350867485,-0.166543350814306,
-1.60050712143809));
#12213=CARTESIAN_POINT('Ctrl Pts',(-0.388626558458099,-0.123401821157026,
-1.59665523941937));
#12214=CARTESIAN_POINT('Ctrl Pts',(-0.397005914195118,-0.07938,-1.59456899932179));
#12215=CARTESIAN_POINT('Origin',(1.11022302462516E-16,-0.07938,-1.675));
#12216=CARTESIAN_POINT('Origin',(0.,-0.07938,0.));
#12217=CARTESIAN_POINT('',(0.846804978391753,-0.07938,-1.40825612658882));
#12218=CARTESIAN_POINT('Origin',(0.,-0.07938,0.));
#12219=CARTESIAN_POINT('Origin',(1.18440385848747,-0.07938,-1.18440385848747));
#12220=CARTESIAN_POINT('Origin',(1.18440385848747,0.,-1.18440385848747));
#12221=CARTESIAN_POINT('',(1.40825612658882,-0.07938,-0.846804978391753));
#12222=CARTESIAN_POINT('Ctrl Pts',(1.40825612658882,-0.0793800000000001,
-0.846804978391753));
#12223=CARTESIAN_POINT('Ctrl Pts',(1.40380622184538,-0.123401821157026,
-0.854205272175555));
#12224=CARTESIAN_POINT('Ctrl Pts',(1.39550172959303,-0.166543350814306,
-0.867957148219442));
#12225=CARTESIAN_POINT('Ctrl Pts',(1.3735491215176,-0.237231147975234,-0.902193646979983));
#12226=CARTESIAN_POINT('Ctrl Pts',(1.36127834356734,-0.266264900654908,
-0.920778333482565));
#12227=CARTESIAN_POINT('Ctrl Pts',(1.33211611256184,-0.317195968905306,
-0.962485392528369));
#12228=CARTESIAN_POINT('Ctrl Pts',(1.31521005565926,-0.33909093068465,-0.985600426557816));
#12229=CARTESIAN_POINT('Ctrl Pts',(1.27866649102984,-0.373586846396559,
-1.03253285680459));
#12230=CARTESIAN_POINT('Ctrl Pts',(1.25722555095714,-0.388086240756494,
-1.05871835910697));
#12231=CARTESIAN_POINT('Ctrl Pts',(1.2107812086231,-0.407068917407805,-1.11153475808518));
#12232=CARTESIAN_POINT('Ctrl Pts',(1.18575674747573,-0.411552957311693,
-1.13814686046673));
#12233=CARTESIAN_POINT('Ctrl Pts',(1.13814686046673,-0.411552957311693,
-1.18575674747573));
#12234=CARTESIAN_POINT('Ctrl Pts',(1.11153475808518,-0.407068917407805,
-1.2107812086231));
#12235=CARTESIAN_POINT('Ctrl Pts',(1.05871835910697,-0.388086240756494,
-1.25722555095714));
#12236=CARTESIAN_POINT('Ctrl Pts',(1.03253285680459,-0.373586846396559,
-1.27866649102984));
#12237=CARTESIAN_POINT('Ctrl Pts',(0.985600426557816,-0.33909093068465,
-1.31521005565926));
#12238=CARTESIAN_POINT('Ctrl Pts',(0.962485392528369,-0.317195968905306,
-1.33211611256184));
#12239=CARTESIAN_POINT('Ctrl Pts',(0.920778333482565,-0.266264900654909,
-1.36127834356734));
#12240=CARTESIAN_POINT('Ctrl Pts',(0.902193646979983,-0.237231147975234,
-1.3735491215176));
#12241=CARTESIAN_POINT('Ctrl Pts',(0.867957148219442,-0.166543350814306,
-1.39550172959303));
#12242=CARTESIAN_POINT('Ctrl Pts',(0.854205272175555,-0.123401821157026,
-1.40380622184538));
#12243=CARTESIAN_POINT('Ctrl Pts',(0.846804978391753,-0.0793800000000001,
-1.40825612658882));
#12244=CARTESIAN_POINT('Origin',(1.18440385848747,-0.07938,-1.18440385848747));
#12245=CARTESIAN_POINT('Origin',(0.,-0.27783,0.));
#12246=CARTESIAN_POINT('',(-1.643248,-0.47628,2.01239840340529E-16));
#12247=CARTESIAN_POINT('Origin',(0.,-0.47628,0.));
#12248=CARTESIAN_POINT('',(-1.643248,-0.27783,2.01239840340529E-16));
#12249=CARTESIAN_POINT('',(1.59456899932179,-0.07938,0.397005914195118));
#12250=CARTESIAN_POINT('Origin',(0.,-0.07938,0.));
#12251=CARTESIAN_POINT('',(1.59456899932179,-0.07938,-0.397005914195118));
#12252=CARTESIAN_POINT('Ctrl Pts',(1.59456899932179,-0.0793800000000001,
0.397005914195118));
#12253=CARTESIAN_POINT('Ctrl Pts',(1.59665523941937,-0.123401821157026,
0.388626558458099));
#12254=CARTESIAN_POINT('Ctrl Pts',(1.60050712143809,-0.166543350814306,
0.373030350867485));
#12255=CARTESIAN_POINT('Ctrl Pts',(1.60919314384089,-0.237231147975234,
0.333298652394954));
#12256=CARTESIAN_POINT('Ctrl Pts',(1.61365775139403,-0.266264900654909,
0.311480544243686));
#12257=CARTESIAN_POINT('Ctrl Pts',(1.62252828437015,-0.317195968905306,
0.261368388670537));
#12258=CARTESIAN_POINT('Ctrl Pts',(1.62691869420078,-0.33909093068465,0.233069203882014));
#12259=CARTESIAN_POINT('Ctrl Pts',(1.63426473152765,-0.373586846396559,
0.174042761838764));
#12260=CARTESIAN_POINT('Ctrl Pts',(1.63761964365402,-0.388086240756494,
0.140365781471549));
#12261=CARTESIAN_POINT('Ctrl Pts',(1.64212536811722,-0.407068917407805,
0.0701778381840612));
#12262=CARTESIAN_POINT('Ctrl Pts',(1.643248,-0.411552957311693,0.0336652739555916));
#12263=CARTESIAN_POINT('Ctrl Pts',(1.643248,-0.411552957311693,-0.0336652739555916));
#12264=CARTESIAN_POINT('Ctrl Pts',(1.64212536811722,-0.407068917407805,
-0.0701778381840612));
#12265=CARTESIAN_POINT('Ctrl Pts',(1.63761964365402,-0.388086240756494,
-0.140365781471549));
#12266=CARTESIAN_POINT('Ctrl Pts',(1.63426473152765,-0.373586846396559,
-0.174042761838764));
#12267=CARTESIAN_POINT('Ctrl Pts',(1.62691869420078,-0.33909093068465,-0.233069203882014));
#12268=CARTESIAN_POINT('Ctrl Pts',(1.62252828437015,-0.317195968905306,
-0.261368388670537));
#12269=CARTESIAN_POINT('Ctrl Pts',(1.61365775139403,-0.266264900654909,
-0.311480544243686));
#12270=CARTESIAN_POINT('Ctrl Pts',(1.60919314384089,-0.237231147975234,
-0.333298652394954));
#12271=CARTESIAN_POINT('Ctrl Pts',(1.60050712143809,-0.166543350814306,
-0.373030350867485));
#12272=CARTESIAN_POINT('Ctrl Pts',(1.59665523941937,-0.123401821157026,
-0.388626558458099));
#12273=CARTESIAN_POINT('Ctrl Pts',(1.59456899932179,-0.07938,-0.397005914195118));
#12274=CARTESIAN_POINT('Origin',(0.,-0.07938,0.));
#12275=CARTESIAN_POINT('Origin',(0.,-0.07938,0.));
#12276=CARTESIAN_POINT('Origin',(1.675,-0.07938,0.));
#12277=CARTESIAN_POINT('Origin',(1.675,0.,0.));
#12278=CARTESIAN_POINT('Origin',(1.675,-0.07938,0.));
#12279=CARTESIAN_POINT('Origin',(0.,-0.47628,0.));
#12280=CARTESIAN_POINT('Origin',(0.,-0.07938,0.));
#25020=UNCERTAINTY_MEASURE_WITH_UNIT(LENGTH_MEASURE(0.001),#25075,
'DISTANCE_ACCURACY_VALUE',
'Maximum model space distance between geometric entities at asserted c
onnectivities');
#25040=UNCERTAINTY_MEASURE_WITH_UNIT(LENGTH_MEASURE(0.001),#25075,
'DISTANCE_ACCURACY_VALUE',
'Maximum model space distance between geometric entities at asserted c
onnectivities');
#25054=(
GEOMETRIC_REPRESENTATION_CONTEXT(3)
GLOBAL_UNCERTAINTY_ASSIGNED_CONTEXT((#25020))
GLOBAL_UNIT_ASSIGNED_CONTEXT((#25075,#25077,#25078))
REPRESENTATION_CONTEXT('','3D')
);
#25074=(
GEOMETRIC_REPRESENTATION_CONTEXT(3)
GLOBAL_UNCERTAINTY_ASSIGNED_CONTEXT((#25040))
GLOBAL_UNIT_ASSIGNED_CONTEXT((#25075,#25077,#25078))
REPRESENTATION_CONTEXT('','3D')
);
#25075=(
LENGTH_UNIT()
NAMED_UNIT(*)
SI_UNIT(.CENTI.,.METRE.)
);
#25077=(
NAMED_UNIT(*)
PLANE_ANGLE_UNIT()
SI_UNIT($,.RADIAN.)
);
#25078=(
NAMED_UNIT(*)
SI_UNIT($,.STERADIAN.)
SOLID_ANGLE_UNIT()
);
#25092=SHAPE_DEFINITION_REPRESENTATION(#25125,#25207);
#25125=PRODUCT_DEFINITION_SHAPE('',$,#25241);
#25207=SHAPE_REPRESENTATION('',(#8630),#25054);
#25227=PRODUCT_DEFINITION_CONTEXT('part definition',#25328,'design');
#25241=PRODUCT_DEFINITION('Cage','Cage',#25274,#25227);
#25274=PRODUCT_DEFINITION_FORMATION('',$,#25343);
#25328=APPLICATION_CONTEXT(
'Core Data for Automotive Mechanical Design Process');
#25329=PRODUCT_CONTEXT('part definition',#25328,'mechanical');
#25343=PRODUCT('Cage','Cage','Cage',(#25329));
#25433=COLOUR_RGB('Grey',0.48,0.52,0.57);
#25434=FILL_AREA_STYLE_COLOUR('',#25433);
#25435=FILL_AREA_STYLE('',(#25434));
#25436=SURFACE_STYLE_FILL_AREA(#25435);
#25437=SURFACE_SIDE_STYLE('',(#25436));
#25438=SURFACE_STYLE_USAGE(.BOTH.,#25437);
#25439=PRESENTATION_STYLE_ASSIGNMENT((#25438));
ENDSEC;
END-ISO-10303-21;
